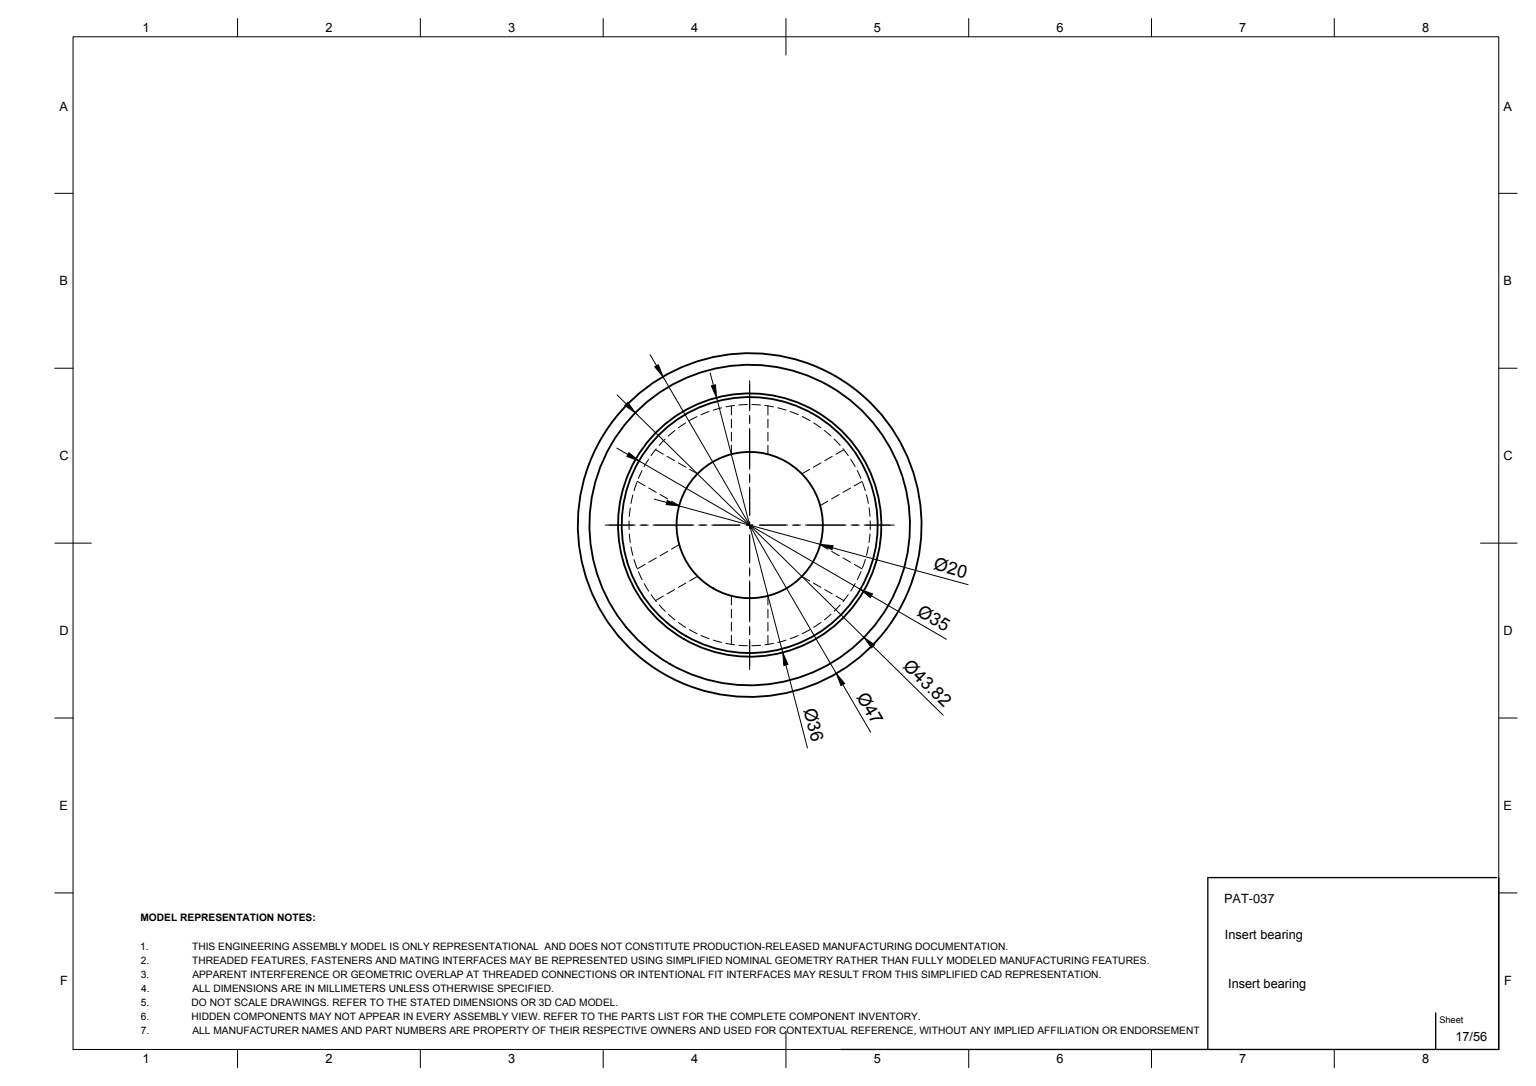
ISO-10303-21;
HEADER;
/* Generated by software containing ST-Developer
 * from STEP Tools, Inc. (www.steptools.com) 
 */

FILE_DESCRIPTION(
/* description */ ('Flywheel Crank-Slider'),
/* implementation_level */ '2;1');

FILE_NAME(
/* name */ 'Insert bearing.step',
/* time_stamp */ '2026-10-28T03:23:13-07:00',
/* author */ (''),
/* organization */ (''),
/* preprocessor_version */ 'ST-DEVELOPER v20.2',
/* originating_system */ 'Autodesk Translation Framework v15.17.0.0',
/* authorisation */ '');

FILE_SCHEMA (('AUTOMOTIVE_DESIGN { 1 0 10303 214 3 1 1 }'));
ENDSEC;

DATA;
#10=MECHANICAL_DESIGN_GEOMETRIC_PRESENTATION_REPRESENTATION('',(#681,#682),#17322);
#457=B_SPLINE_CURVE_WITH_KNOTS('',3,(#14534,#14535,#14536,#14537,#14538,
#14539,#14540,#14541,#14542,#14543),.UNSPECIFIED.,.F.,.F.,(4,2,2,2,4),(1.13193471301885,
1.22626174930539,1.32058878559194,1.41491753480854,1.50924628402513),
 .UNSPECIFIED.);
#458=B_SPLINE_CURVE_WITH_KNOTS('',3,(#14545,#14546,#14547,#14548,#14549,
#14550,#14551,#14552,#14553,#14554,#14555,#14556,#14557,#14558,#14559,#14560,
#14561,#14562),.UNSPECIFIED.,.F.,.F.,(4,2,2,2,2,2,2,2,4),(0.377311571006283,
0.471638607292829,0.565965643579376,0.66029439279597,0.754623142012565,
0.84895189122916,0.943280640445754,1.0376076767323,1.13193471301885),
 .UNSPECIFIED.);
#459=B_SPLINE_CURVE_WITH_KNOTS('',3,(#14563,#14564,#14565,#14566,#14567,
#14568,#14569,#14570,#14571,#14572),.UNSPECIFIED.,.F.,.F.,(4,2,2,2,4),(1.50924628402513,
1.60357503324173,1.69790378245832,1.79223081874487,1.88655785503141),
 .UNSPECIFIED.);
#460=B_SPLINE_CURVE_WITH_KNOTS('',3,(#14575,#14576,#14577,#14578,#14579,
#14580,#14581,#14582,#14583,#14584,#14585,#14586,#14587,#14588,#14589,#14590,
#14591,#14592,#14593,#14594,#14595,#14596,#14597,#14598,#14599,#14600,#14601,
#14602,#14603,#14604,#14605,#14606,#14607,#14608),.UNSPECIFIED.,.T.,.F.,
(4,2,2,2,2,2,2,2,2,2,2,2,2,2,2,2,4),(0.,0.0946120580087934,0.189224116017587,
0.283822945575014,0.378421775132442,0.47302060468987,0.567619434247297,
0.662231492256091,0.756843550264884,0.851455608273677,0.94606766628247,
1.0406664958399,1.13526532539733,1.22986415495475,1.32446298451218,1.41907504252097,
1.51368710052977),.UNSPECIFIED.);
#461=B_SPLINE_CURVE_WITH_KNOTS('',3,(#14611,#14612,#14613,#14614,#14615,
#14616,#14617,#14618,#14619,#14620,#14621,#14622,#14623,#14624,#14625,#14626,
#14627,#14628,#14629,#14630,#14631,#14632,#14633,#14634,#14635,#14636,#14637,
#14638,#14639,#14640,#14641,#14642,#14643,#14644),.UNSPECIFIED.,.T.,.F.,
(4,2,2,2,2,2,2,2,2,2,2,2,2,2,2,2,4),(0.,0.0946120580087934,0.189224116017587,
0.283822945575014,0.378421775132442,0.47302060468987,0.567619434247297,
0.66223149225609,0.756843550264884,0.851455608273677,0.94606766628247,1.0406664958399,
1.13526532539733,1.22986415495475,1.32446298451218,1.41907504252097,1.51368710052977),
 .UNSPECIFIED.);
#462=B_SPLINE_CURVE_WITH_KNOTS('',3,(#14648,#14649,#14650,#14651,#14652,
#14653,#14654,#14655,#14656,#14657),.UNSPECIFIED.,.F.,.F.,(4,2,2,2,4),(1.13193471301885,
1.22626174930539,1.32058878559194,1.41491753480854,1.50924628402513),
 .UNSPECIFIED.);
#463=B_SPLINE_CURVE_WITH_KNOTS('',3,(#14659,#14660,#14661,#14662,#14663,
#14664,#14665,#14666,#14667,#14668,#14669,#14670,#14671,#14672,#14673,#14674,
#14675,#14676),.UNSPECIFIED.,.F.,.F.,(4,2,2,2,2,2,2,2,4),(0.377311571006283,
0.47163860729283,0.565965643579376,0.660294392795971,0.754623142012565,
0.84895189122916,0.943280640445755,1.0376076767323,1.13193471301885),
 .UNSPECIFIED.);
#464=B_SPLINE_CURVE_WITH_KNOTS('',3,(#14677,#14678,#14679,#14680,#14681,
#14682,#14683,#14684,#14685,#14686),.UNSPECIFIED.,.F.,.F.,(4,2,2,2,4),(1.50924628402513,
1.60357503324173,1.69790378245832,1.79223081874487,1.88655785503141),
 .UNSPECIFIED.);
#465=B_SPLINE_CURVE_WITH_KNOTS('',3,(#14695,#14696,#14697,#14698,#14699,
#14700,#14701,#14702,#14703,#14704,#14705,#14706,#14707,#14708,#14709,#14710,
#14711,#14712),.UNSPECIFIED.,.F.,.F.,(4,2,2,2,2,2,2,2,4),(0.377311571006282,
0.471638607292829,0.565965643579376,0.660294392795971,0.754623142012565,
0.84895189122916,0.943280640445754,1.0376076767323,1.13193471301885),
 .UNSPECIFIED.);
#466=B_SPLINE_CURVE_WITH_KNOTS('',3,(#14714,#14715,#14716,#14717,#14718,
#14719,#14720,#14721,#14722,#14723),.UNSPECIFIED.,.F.,.F.,(4,2,2,2,4),(1.13193471301885,
1.22626174930539,1.32058878559194,1.41491753480854,1.50924628402513),
 .UNSPECIFIED.);
#467=B_SPLINE_CURVE_WITH_KNOTS('',3,(#14724,#14725,#14726,#14727,#14728,
#14729,#14730,#14731,#14732,#14733),.UNSPECIFIED.,.F.,.F.,(4,2,2,2,4),(1.50924628402513,
1.60357503324172,1.69790378245832,1.79223081874487,1.88655785503141),
 .UNSPECIFIED.);
#468=B_SPLINE_CURVE_WITH_KNOTS('',3,(#14736,#14737,#14738,#14739,#14740,
#14741,#14742,#14743,#14744,#14745,#14746,#14747,#14748,#14749,#14750,#14751,
#14752,#14753),.UNSPECIFIED.,.F.,.F.,(4,2,2,2,2,2,2,2,4),(0.377311571006283,
0.47163860729283,0.565965643579376,0.660294392795971,0.754623142012565,
0.84895189122916,0.943280640445754,1.0376076767323,1.13193471301885),
 .UNSPECIFIED.);
#469=B_SPLINE_CURVE_WITH_KNOTS('',3,(#14755,#14756,#14757,#14758,#14759,
#14760,#14761,#14762,#14763,#14764),.UNSPECIFIED.,.F.,.F.,(4,2,2,2,4),(1.13193471301885,
1.22626174930539,1.32058878559194,1.41491753480854,1.50924628402513),
 .UNSPECIFIED.);
#470=B_SPLINE_CURVE_WITH_KNOTS('',3,(#14765,#14766,#14767,#14768,#14769,
#14770,#14771,#14772,#14773,#14774),.UNSPECIFIED.,.F.,.F.,(4,2,2,2,4),(1.50924628402513,
1.60357503324173,1.69790378245832,1.79223081874487,1.88655785503141),
 .UNSPECIFIED.);
#471=B_SPLINE_CURVE_WITH_KNOTS('',3,(#14777,#14778,#14779,#14780,#14781,
#14782,#14783,#14784,#14785,#14786,#14787,#14788,#14789,#14790,#14791,#14792,
#14793,#14794),.UNSPECIFIED.,.F.,.F.,(4,2,2,2,2,2,2,2,4),(0.377311571006282,
0.471638607292829,0.565965643579376,0.66029439279597,0.754623142012565,
0.84895189122916,0.943280640445754,1.0376076767323,1.13193471301885),
 .UNSPECIFIED.);
#472=B_SPLINE_CURVE_WITH_KNOTS('',3,(#14796,#14797,#14798,#14799,#14800,
#14801,#14802,#14803,#14804,#14805),.UNSPECIFIED.,.F.,.F.,(4,2,2,2,4),(1.13193471301885,
1.22626174930539,1.32058878559194,1.41491753480854,1.50924628402513),
 .UNSPECIFIED.);
#473=B_SPLINE_CURVE_WITH_KNOTS('',3,(#14806,#14807,#14808,#14809,#14810,
#14811,#14812,#14813,#14814,#14815),.UNSPECIFIED.,.F.,.F.,(4,2,2,2,4),(1.50924628402513,
1.60357503324172,1.69790378245832,1.79223081874487,1.88655785503141),
 .UNSPECIFIED.);
#474=B_SPLINE_CURVE_WITH_KNOTS('',3,(#14818,#14819,#14820,#14821,#14822,
#14823,#14824,#14825,#14826,#14827,#14828,#14829,#14830,#14831,#14832,#14833,
#14834,#14835),.UNSPECIFIED.,.F.,.F.,(4,2,2,2,2,2,2,2,4),(0.377311571006283,
0.471638607292829,0.565965643579376,0.660294392795971,0.754623142012565,
0.84895189122916,0.943280640445755,1.0376076767323,1.13193471301885),
 .UNSPECIFIED.);
#475=B_SPLINE_CURVE_WITH_KNOTS('',3,(#14837,#14838,#14839,#14840,#14841,
#14842,#14843,#14844,#14845,#14846),.UNSPECIFIED.,.F.,.F.,(4,2,2,2,4),(1.13193471301885,
1.22626174930539,1.32058878559194,1.41491753480854,1.50924628402513),
 .UNSPECIFIED.);
#476=B_SPLINE_CURVE_WITH_KNOTS('',3,(#14847,#14848,#14849,#14850,#14851,
#14852,#14853,#14854,#14855,#14856),.UNSPECIFIED.,.F.,.F.,(4,2,2,2,4),(1.50924628402513,
1.60357503324172,1.69790378245832,1.79223081874487,1.88655785503141),
 .UNSPECIFIED.);
#477=B_SPLINE_CURVE_WITH_KNOTS('',3,(#14860,#14861,#14862,#14863,#14864,
#14865,#14866,#14867,#14868,#14869,#14870,#14871,#14872,#14873,#14874,#14875,
#14876,#14877,#14878,#14879,#14880,#14881,#14882,#14883,#14884,#14885,#14886,
#14887,#14888,#14889,#14890,#14891,#14892,#14893),.UNSPECIFIED.,.T.,.F.,
(4,2,2,2,2,2,2,2,2,2,2,2,2,2,2,2,4),(0.,0.0946120580087934,0.189224116017587,
0.283822945575014,0.378421775132442,0.47302060468987,0.567619434247297,
0.66223149225609,0.756843550264884,0.851455608273677,0.94606766628247,1.0406664958399,
1.13526532539733,1.22986415495475,1.32446298451218,1.41907504252097,1.51368710052977),
 .UNSPECIFIED.);
#478=B_SPLINE_CURVE_WITH_KNOTS('',3,(#14896,#14897,#14898,#14899,#14900,
#14901,#14902,#14903,#14904,#14905,#14906,#14907,#14908,#14909,#14910,#14911,
#14912,#14913,#14914,#14915,#14916,#14917,#14918,#14919,#14920,#14921,#14922,
#14923,#14924,#14925,#14926,#14927,#14928,#14929),.UNSPECIFIED.,.T.,.F.,
(4,2,2,2,2,2,2,2,2,2,2,2,2,2,2,2,4),(0.,0.0946120580087934,0.189224116017587,
0.283822945575014,0.378421775132442,0.47302060468987,0.567619434247297,
0.66223149225609,0.756843550264884,0.851455608273677,0.94606766628247,1.0406664958399,
1.13526532539733,1.22986415495475,1.32446298451218,1.41907504252097,1.51368710052977),
 .UNSPECIFIED.);
#479=B_SPLINE_CURVE_WITH_KNOTS('',3,(#14934,#14935,#14936,#14937,#14938,
#14939,#14940,#14941,#14942,#14943,#14944,#14945,#14946,#14947,#14948,#14949,
#14950,#14951,#14952,#14953,#14954,#14955,#14956,#14957,#14958,#14959,#14960,
#14961,#14962,#14963,#14964,#14965,#14966,#14967),.UNSPECIFIED.,.T.,.F.,
(4,2,2,2,2,2,2,2,2,2,2,2,2,2,2,2,4),(0.,0.0946120580087934,0.189224116017587,
0.283822945575014,0.378421775132442,0.47302060468987,0.567619434247297,
0.66223149225609,0.756843550264884,0.851455608273677,0.94606766628247,1.0406664958399,
1.13526532539733,1.22986415495475,1.32446298451218,1.41907504252097,1.51368710052977),
 .UNSPECIFIED.);
#480=B_SPLINE_CURVE_WITH_KNOTS('',3,(#14970,#14971,#14972,#14973,#14974,
#14975,#14976,#14977,#14978,#14979,#14980,#14981,#14982,#14983,#14984,#14985,
#14986,#14987,#14988,#14989,#14990,#14991,#14992,#14993,#14994,#14995,#14996,
#14997,#14998,#14999,#15000,#15001,#15002,#15003),.UNSPECIFIED.,.T.,.F.,
(4,2,2,2,2,2,2,2,2,2,2,2,2,2,2,2,4),(0.,0.0946120580087934,0.189224116017587,
0.283822945575014,0.378421775132442,0.47302060468987,0.567619434247297,
0.66223149225609,0.756843550264884,0.851455608273677,0.94606766628247,1.0406664958399,
1.13526532539733,1.22986415495475,1.32446298451218,1.41907504252097,1.51368710052977),
 .UNSPECIFIED.);
#512=SPHERICAL_SURFACE('',#10020,2.35);
#577=SHAPE_REPRESENTATION_RELATIONSHIP('SRR','None',#17574,#629);
#629=ADVANCED_BREP_SHAPE_REPRESENTATION('',(#741,#742),#17278);
#681=STYLED_ITEM('',(#17931),#741);
#682=STYLED_ITEM('',(#17931),#742);
#741=MANIFOLD_SOLID_BREP('Body1',#9060);
#742=MANIFOLD_SOLID_BREP('Body2',#9061);
#872=FACE_BOUND('',#2118,.T.);
#873=FACE_BOUND('',#2120,.T.);
#874=FACE_BOUND('',#2121,.T.);
#875=FACE_BOUND('',#2123,.T.);
#876=FACE_BOUND('',#2127,.T.);
#877=FACE_BOUND('',#2128,.T.);
#878=FACE_BOUND('',#2129,.T.);
#879=FACE_BOUND('',#2130,.T.);
#880=FACE_BOUND('',#2131,.T.);
#881=FACE_BOUND('',#2132,.T.);
#882=FACE_BOUND('',#2138,.T.);
#883=FACE_BOUND('',#2140,.T.);
#884=FACE_BOUND('',#2143,.T.);
#885=FACE_BOUND('',#2145,.T.);
#886=FACE_BOUND('',#2146,.T.);
#887=FACE_BOUND('',#2147,.T.);
#888=FACE_BOUND('',#2148,.T.);
#889=FACE_BOUND('',#2149,.T.);
#890=FACE_BOUND('',#2150,.T.);
#1115=PLANE('',#10018);
#1116=PLANE('',#10023);
#1117=PLANE('',#10033);
#1118=PLANE('',#10035);
#1119=PLANE('',#10039);
#1494=FACE_OUTER_BOUND('',#2116,.T.);
#1495=FACE_OUTER_BOUND('',#2117,.T.);
#1496=FACE_OUTER_BOUND('',#2119,.T.);
#1497=FACE_OUTER_BOUND('',#2122,.T.);
#1498=FACE_OUTER_BOUND('',#2124,.T.);
#1499=FACE_OUTER_BOUND('',#2125,.T.);
#1500=FACE_OUTER_BOUND('',#2126,.T.);
#1501=FACE_OUTER_BOUND('',#2133,.T.);
#1502=FACE_OUTER_BOUND('',#2134,.T.);
#1503=FACE_OUTER_BOUND('',#2135,.T.);
#1504=FACE_OUTER_BOUND('',#2136,.T.);
#1505=FACE_OUTER_BOUND('',#2137,.T.);
#1506=FACE_OUTER_BOUND('',#2139,.T.);
#1507=FACE_OUTER_BOUND('',#2141,.T.);
#1508=FACE_OUTER_BOUND('',#2142,.T.);
#1509=FACE_OUTER_BOUND('',#2144,.T.);
#2116=EDGE_LOOP('',(#6840,#6841,#6842,#6843));
#2117=EDGE_LOOP('',(#6844));
#2118=EDGE_LOOP('',(#6845));
#2119=EDGE_LOOP('',(#6846,#6847));
#2120=EDGE_LOOP('',(#6848));
#2121=EDGE_LOOP('',(#6849));
#2122=EDGE_LOOP('',(#6850));
#2123=EDGE_LOOP('',(#6851));
#2124=EDGE_LOOP('',(#6852,#6853,#6854,#6855,#6856,#6857));
#2125=EDGE_LOOP('',(#6858,#6859,#6860,#6861,#6862,#6863));
#2126=EDGE_LOOP('',(#6864,#6865,#6866,#6867));
#2127=EDGE_LOOP('',(#6868,#6869,#6870));
#2128=EDGE_LOOP('',(#6871,#6872,#6873));
#2129=EDGE_LOOP('',(#6874,#6875,#6876));
#2130=EDGE_LOOP('',(#6877,#6878,#6879));
#2131=EDGE_LOOP('',(#6880,#6881,#6882));
#2132=EDGE_LOOP('',(#6883,#6884,#6885));
#2133=EDGE_LOOP('',(#6886,#6887,#6888,#6889,#6890,#6891));
#2134=EDGE_LOOP('',(#6892,#6893,#6894,#6895,#6896,#6897));
#2135=EDGE_LOOP('',(#6898,#6899,#6900,#6901,#6902,#6903));
#2136=EDGE_LOOP('',(#6904,#6905,#6906,#6907,#6908,#6909));
#2137=EDGE_LOOP('',(#6910));
#2138=EDGE_LOOP('',(#6911));
#2139=EDGE_LOOP('',(#6912));
#2140=EDGE_LOOP('',(#6913));
#2141=EDGE_LOOP('',(#6914,#6915,#6916,#6917));
#2142=EDGE_LOOP('',(#6918));
#2143=EDGE_LOOP('',(#6919));
#2144=EDGE_LOOP('',(#6920,#6921,#6922,#6923));
#2145=EDGE_LOOP('',(#6924));
#2146=EDGE_LOOP('',(#6925));
#2147=EDGE_LOOP('',(#6926));
#2148=EDGE_LOOP('',(#6927));
#2149=EDGE_LOOP('',(#6928));
#2150=EDGE_LOOP('',(#6929));
#2836=LINE('',#14519,#3447);
#2837=LINE('',#14574,#3448);
#2838=LINE('',#14646,#3449);
#2839=LINE('',#14691,#3450);
#2840=LINE('',#14859,#3451);
#2841=LINE('',#14930,#3452);
#2842=LINE('',#14933,#3453);
#2843=LINE('',#15004,#3454);
#2844=LINE('',#15014,#3455);
#2845=LINE('',#15019,#3456);
#3447=VECTOR('',#11714,1.8);
#3448=VECTOR('',#11731,0.25);
#3449=VECTOR('',#11734,0.25);
#3450=VECTOR('',#11739,1.65);
#3451=VECTOR('',#11744,0.25);
#3452=VECTOR('',#11747,0.25);
#3453=VECTOR('',#11750,0.25);
#3454=VECTOR('',#11753,0.25);
#3455=VECTOR('',#11766,1.75);
#3456=VECTOR('',#11773,1.);
#3977=CIRCLE('',#10016,1.8);
#3978=CIRCLE('',#10017,1.8);
#3979=CIRCLE('',#10019,2.19089023002066);
#3980=CIRCLE('',#10021,2.35);
#3981=CIRCLE('',#10022,2.19089023002066);
#3982=CIRCLE('',#10027,1.65);
#3983=CIRCLE('',#10028,1.65);
#3984=CIRCLE('',#10034,1.);
#3985=CIRCLE('',#10036,1.75);
#3986=CIRCLE('',#10038,1.75);
#3987=CIRCLE('',#10040,1.);
#4511=VERTEX_POINT('',#14516);
#4512=VERTEX_POINT('',#14518);
#4513=VERTEX_POINT('',#14522);
#4514=VERTEX_POINT('',#14525);
#4515=VERTEX_POINT('',#14526);
#4516=VERTEX_POINT('',#14528);
#4517=VERTEX_POINT('',#14532);
#4518=VERTEX_POINT('',#14533);
#4519=VERTEX_POINT('',#14544);
#4520=VERTEX_POINT('',#14573);
#4521=VERTEX_POINT('',#14610);
#4522=VERTEX_POINT('',#14645);
#4523=VERTEX_POINT('',#14647);
#4524=VERTEX_POINT('',#14658);
#4525=VERTEX_POINT('',#14688);
#4526=VERTEX_POINT('',#14690);
#4527=VERTEX_POINT('',#14693);
#4528=VERTEX_POINT('',#14694);
#4529=VERTEX_POINT('',#14713);
#4530=VERTEX_POINT('',#14734);
#4531=VERTEX_POINT('',#14735);
#4532=VERTEX_POINT('',#14754);
#4533=VERTEX_POINT('',#14775);
#4534=VERTEX_POINT('',#14776);
#4535=VERTEX_POINT('',#14795);
#4536=VERTEX_POINT('',#14816);
#4537=VERTEX_POINT('',#14817);
#4538=VERTEX_POINT('',#14836);
#4539=VERTEX_POINT('',#14858);
#4540=VERTEX_POINT('',#14895);
#4541=VERTEX_POINT('',#14932);
#4542=VERTEX_POINT('',#14969);
#4543=VERTEX_POINT('',#15006);
#4544=VERTEX_POINT('',#15009);
#4545=VERTEX_POINT('',#15012);
#4546=VERTEX_POINT('',#15016);
#5377=EDGE_CURVE('',#4511,#4511,#3977,.T.);
#5378=EDGE_CURVE('',#4511,#4512,#2836,.T.);
#5379=EDGE_CURVE('',#4512,#4512,#3978,.T.);
#5380=EDGE_CURVE('',#4513,#4513,#3979,.T.);
#5381=EDGE_CURVE('',#4514,#4515,#3980,.T.);
#5382=EDGE_CURVE('',#4516,#4516,#3981,.T.);
#5383=EDGE_CURVE('',#4517,#4518,#457,.T.);
#5384=EDGE_CURVE('',#4519,#4517,#458,.T.);
#5385=EDGE_CURVE('',#4518,#4519,#459,.T.);
#5386=EDGE_CURVE('',#4518,#4520,#2837,.T.);
#5387=EDGE_CURVE('',#4520,#4520,#460,.T.);
#5388=EDGE_CURVE('',#4521,#4521,#461,.T.);
#5389=EDGE_CURVE('',#4521,#4522,#2838,.T.);
#5390=EDGE_CURVE('',#4523,#4522,#462,.T.);
#5391=EDGE_CURVE('',#4524,#4523,#463,.T.);
#5392=EDGE_CURVE('',#4522,#4524,#464,.T.);
#5393=EDGE_CURVE('',#4525,#4525,#3982,.T.);
#5394=EDGE_CURVE('',#4525,#4526,#2839,.T.);
#5395=EDGE_CURVE('',#4526,#4526,#3983,.T.);
#5396=EDGE_CURVE('',#4527,#4528,#465,.T.);
#5397=EDGE_CURVE('',#4528,#4529,#466,.T.);
#5398=EDGE_CURVE('',#4529,#4527,#467,.T.);
#5399=EDGE_CURVE('',#4530,#4531,#468,.T.);
#5400=EDGE_CURVE('',#4531,#4532,#469,.T.);
#5401=EDGE_CURVE('',#4532,#4530,#470,.T.);
#5402=EDGE_CURVE('',#4533,#4534,#471,.T.);
#5403=EDGE_CURVE('',#4534,#4535,#472,.T.);
#5404=EDGE_CURVE('',#4535,#4533,#473,.T.);
#5405=EDGE_CURVE('',#4536,#4537,#474,.T.);
#5406=EDGE_CURVE('',#4537,#4538,#475,.T.);
#5407=EDGE_CURVE('',#4538,#4536,#476,.T.);
#5408=EDGE_CURVE('',#4529,#4539,#2840,.T.);
#5409=EDGE_CURVE('',#4539,#4539,#477,.T.);
#5410=EDGE_CURVE('',#4540,#4540,#478,.T.);
#5411=EDGE_CURVE('',#4540,#4532,#2841,.T.);
#5412=EDGE_CURVE('',#4535,#4541,#2842,.T.);
#5413=EDGE_CURVE('',#4541,#4541,#479,.T.);
#5414=EDGE_CURVE('',#4542,#4542,#480,.T.);
#5415=EDGE_CURVE('',#4542,#4538,#2843,.T.);
#5416=EDGE_CURVE('',#4543,#4543,#3984,.T.);
#5417=EDGE_CURVE('',#4544,#4544,#3985,.T.);
#5418=EDGE_CURVE('',#4545,#4545,#3986,.T.);
#5419=EDGE_CURVE('',#4545,#4544,#2844,.T.);
#5420=EDGE_CURVE('',#4546,#4546,#3987,.T.);
#5421=EDGE_CURVE('',#4546,#4543,#2845,.T.);
#6840=ORIENTED_EDGE('',*,*,#5377,.T.);
#6841=ORIENTED_EDGE('',*,*,#5378,.T.);
#6842=ORIENTED_EDGE('',*,*,#5379,.F.);
#6843=ORIENTED_EDGE('',*,*,#5378,.F.);
#6844=ORIENTED_EDGE('',*,*,#5380,.F.);
#6845=ORIENTED_EDGE('',*,*,#5379,.T.);
#6846=ORIENTED_EDGE('',*,*,#5381,.T.);
#6847=ORIENTED_EDGE('',*,*,#5381,.F.);
#6848=ORIENTED_EDGE('',*,*,#5380,.T.);
#6849=ORIENTED_EDGE('',*,*,#5382,.F.);
#6850=ORIENTED_EDGE('',*,*,#5382,.T.);
#6851=ORIENTED_EDGE('',*,*,#5377,.F.);
#6852=ORIENTED_EDGE('',*,*,#5383,.F.);
#6853=ORIENTED_EDGE('',*,*,#5384,.F.);
#6854=ORIENTED_EDGE('',*,*,#5385,.F.);
#6855=ORIENTED_EDGE('',*,*,#5386,.T.);
#6856=ORIENTED_EDGE('',*,*,#5387,.F.);
#6857=ORIENTED_EDGE('',*,*,#5386,.F.);
#6858=ORIENTED_EDGE('',*,*,#5388,.F.);
#6859=ORIENTED_EDGE('',*,*,#5389,.T.);
#6860=ORIENTED_EDGE('',*,*,#5390,.F.);
#6861=ORIENTED_EDGE('',*,*,#5391,.F.);
#6862=ORIENTED_EDGE('',*,*,#5392,.F.);
#6863=ORIENTED_EDGE('',*,*,#5389,.F.);
#6864=ORIENTED_EDGE('',*,*,#5393,.F.);
#6865=ORIENTED_EDGE('',*,*,#5394,.T.);
#6866=ORIENTED_EDGE('',*,*,#5395,.T.);
#6867=ORIENTED_EDGE('',*,*,#5394,.F.);
#6868=ORIENTED_EDGE('',*,*,#5384,.T.);
#6869=ORIENTED_EDGE('',*,*,#5383,.T.);
#6870=ORIENTED_EDGE('',*,*,#5385,.T.);
#6871=ORIENTED_EDGE('',*,*,#5391,.T.);
#6872=ORIENTED_EDGE('',*,*,#5390,.T.);
#6873=ORIENTED_EDGE('',*,*,#5392,.T.);
#6874=ORIENTED_EDGE('',*,*,#5396,.T.);
#6875=ORIENTED_EDGE('',*,*,#5397,.T.);
#6876=ORIENTED_EDGE('',*,*,#5398,.T.);
#6877=ORIENTED_EDGE('',*,*,#5399,.T.);
#6878=ORIENTED_EDGE('',*,*,#5400,.T.);
#6879=ORIENTED_EDGE('',*,*,#5401,.T.);
#6880=ORIENTED_EDGE('',*,*,#5402,.T.);
#6881=ORIENTED_EDGE('',*,*,#5403,.T.);
#6882=ORIENTED_EDGE('',*,*,#5404,.T.);
#6883=ORIENTED_EDGE('',*,*,#5405,.T.);
#6884=ORIENTED_EDGE('',*,*,#5406,.T.);
#6885=ORIENTED_EDGE('',*,*,#5407,.T.);
#6886=ORIENTED_EDGE('',*,*,#5397,.F.);
#6887=ORIENTED_EDGE('',*,*,#5396,.F.);
#6888=ORIENTED_EDGE('',*,*,#5398,.F.);
#6889=ORIENTED_EDGE('',*,*,#5408,.T.);
#6890=ORIENTED_EDGE('',*,*,#5409,.F.);
#6891=ORIENTED_EDGE('',*,*,#5408,.F.);
#6892=ORIENTED_EDGE('',*,*,#5410,.F.);
#6893=ORIENTED_EDGE('',*,*,#5411,.T.);
#6894=ORIENTED_EDGE('',*,*,#5400,.F.);
#6895=ORIENTED_EDGE('',*,*,#5399,.F.);
#6896=ORIENTED_EDGE('',*,*,#5401,.F.);
#6897=ORIENTED_EDGE('',*,*,#5411,.F.);
#6898=ORIENTED_EDGE('',*,*,#5403,.F.);
#6899=ORIENTED_EDGE('',*,*,#5402,.F.);
#6900=ORIENTED_EDGE('',*,*,#5404,.F.);
#6901=ORIENTED_EDGE('',*,*,#5412,.T.);
#6902=ORIENTED_EDGE('',*,*,#5413,.F.);
#6903=ORIENTED_EDGE('',*,*,#5412,.F.);
#6904=ORIENTED_EDGE('',*,*,#5414,.F.);
#6905=ORIENTED_EDGE('',*,*,#5415,.T.);
#6906=ORIENTED_EDGE('',*,*,#5406,.F.);
#6907=ORIENTED_EDGE('',*,*,#5405,.F.);
#6908=ORIENTED_EDGE('',*,*,#5407,.F.);
#6909=ORIENTED_EDGE('',*,*,#5415,.F.);
#6910=ORIENTED_EDGE('',*,*,#5395,.F.);
#6911=ORIENTED_EDGE('',*,*,#5416,.T.);
#6912=ORIENTED_EDGE('',*,*,#5417,.F.);
#6913=ORIENTED_EDGE('',*,*,#5393,.T.);
#6914=ORIENTED_EDGE('',*,*,#5418,.F.);
#6915=ORIENTED_EDGE('',*,*,#5419,.T.);
#6916=ORIENTED_EDGE('',*,*,#5417,.T.);
#6917=ORIENTED_EDGE('',*,*,#5419,.F.);
#6918=ORIENTED_EDGE('',*,*,#5418,.T.);
#6919=ORIENTED_EDGE('',*,*,#5420,.F.);
#6920=ORIENTED_EDGE('',*,*,#5420,.T.);
#6921=ORIENTED_EDGE('',*,*,#5421,.T.);
#6922=ORIENTED_EDGE('',*,*,#5416,.F.);
#6923=ORIENTED_EDGE('',*,*,#5421,.F.);
#6924=ORIENTED_EDGE('',*,*,#5388,.T.);
#6925=ORIENTED_EDGE('',*,*,#5387,.T.);
#6926=ORIENTED_EDGE('',*,*,#5410,.T.);
#6927=ORIENTED_EDGE('',*,*,#5409,.T.);
#6928=ORIENTED_EDGE('',*,*,#5414,.T.);
#6929=ORIENTED_EDGE('',*,*,#5413,.T.);
#8395=CYLINDRICAL_SURFACE('',#10015,1.8);
#8396=CYLINDRICAL_SURFACE('',#10024,0.25);
#8397=CYLINDRICAL_SURFACE('',#10025,0.25);
#8398=CYLINDRICAL_SURFACE('',#10026,1.65);
#8399=CYLINDRICAL_SURFACE('',#10029,0.25);
#8400=CYLINDRICAL_SURFACE('',#10030,0.25);
#8401=CYLINDRICAL_SURFACE('',#10031,0.25);
#8402=CYLINDRICAL_SURFACE('',#10032,0.25);
#8403=CYLINDRICAL_SURFACE('',#10037,1.75);
#8404=CYLINDRICAL_SURFACE('',#10041,1.);
#8685=ADVANCED_FACE('',(#1494),#8395,.F.);
#8686=ADVANCED_FACE('',(#1495,#872),#1115,.T.);
#8687=ADVANCED_FACE('',(#1496,#873,#874),#512,.T.);
#8688=ADVANCED_FACE('',(#1497,#875),#1116,.T.);
#8689=ADVANCED_FACE('',(#1498),#8396,.F.);
#8690=ADVANCED_FACE('',(#1499),#8397,.F.);
#8691=ADVANCED_FACE('',(#1500,#876,#877,#878,#879,#880,#881),#8398,.T.);
#8692=ADVANCED_FACE('',(#1501),#8399,.F.);
#8693=ADVANCED_FACE('',(#1502),#8400,.F.);
#8694=ADVANCED_FACE('',(#1503),#8401,.F.);
#8695=ADVANCED_FACE('',(#1504),#8402,.F.);
#8696=ADVANCED_FACE('',(#1505,#882),#1117,.T.);
#8697=ADVANCED_FACE('',(#1506,#883),#1118,.T.);
#8698=ADVANCED_FACE('',(#1507),#8403,.T.);
#8699=ADVANCED_FACE('',(#1508,#884),#1119,.T.);
#8700=ADVANCED_FACE('',(#1509,#885,#886,#887,#888,#889,#890),#8404,.F.);
#9060=CLOSED_SHELL('',(#8685,#8686,#8687,#8688));
#9061=CLOSED_SHELL('',(#8689,#8690,#8691,#8692,#8693,#8694,#8695,#8696,
#8697,#8698,#8699,#8700));
#10014=AXIS2_PLACEMENT_3D('',#14514,#11708,#11709);
#10015=AXIS2_PLACEMENT_3D('',#14515,#11710,#11711);
#10016=AXIS2_PLACEMENT_3D('',#14517,#11712,#11713);
#10017=AXIS2_PLACEMENT_3D('',#14520,#11715,#11716);
#10018=AXIS2_PLACEMENT_3D('',#14521,#11717,#11718);
#10019=AXIS2_PLACEMENT_3D('',#14523,#11719,#11720);
#10020=AXIS2_PLACEMENT_3D('',#14524,#11721,#11722);
#10021=AXIS2_PLACEMENT_3D('',#14527,#11723,#11724);
#10022=AXIS2_PLACEMENT_3D('',#14529,#11725,#11726);
#10023=AXIS2_PLACEMENT_3D('',#14530,#11727,#11728);
#10024=AXIS2_PLACEMENT_3D('',#14531,#11729,#11730);
#10025=AXIS2_PLACEMENT_3D('',#14609,#11732,#11733);
#10026=AXIS2_PLACEMENT_3D('',#14687,#11735,#11736);
#10027=AXIS2_PLACEMENT_3D('',#14689,#11737,#11738);
#10028=AXIS2_PLACEMENT_3D('',#14692,#11740,#11741);
#10029=AXIS2_PLACEMENT_3D('',#14857,#11742,#11743);
#10030=AXIS2_PLACEMENT_3D('',#14894,#11745,#11746);
#10031=AXIS2_PLACEMENT_3D('',#14931,#11748,#11749);
#10032=AXIS2_PLACEMENT_3D('',#14968,#11751,#11752);
#10033=AXIS2_PLACEMENT_3D('',#15005,#11754,#11755);
#10034=AXIS2_PLACEMENT_3D('',#15007,#11756,#11757);
#10035=AXIS2_PLACEMENT_3D('',#15008,#11758,#11759);
#10036=AXIS2_PLACEMENT_3D('',#15010,#11760,#11761);
#10037=AXIS2_PLACEMENT_3D('',#15011,#11762,#11763);
#10038=AXIS2_PLACEMENT_3D('',#15013,#11764,#11765);
#10039=AXIS2_PLACEMENT_3D('',#15015,#11767,#11768);
#10040=AXIS2_PLACEMENT_3D('',#15017,#11769,#11770);
#10041=AXIS2_PLACEMENT_3D('',#15018,#11771,#11772);
#11708=DIRECTION('axis',(0.,0.,1.));
#11709=DIRECTION('refdir',(1.,0.,0.));
#11710=DIRECTION('center_axis',(0.,-1.,0.));
#11711=DIRECTION('ref_axis',(1.,0.,0.));
#11712=DIRECTION('center_axis',(0.,-1.,0.));
#11713=DIRECTION('ref_axis',(1.,0.,0.));
#11714=DIRECTION('',(0.,1.,0.));
#11715=DIRECTION('center_axis',(0.,-1.,0.));
#11716=DIRECTION('ref_axis',(1.,0.,0.));
#11717=DIRECTION('center_axis',(0.,1.,0.));
#11718=DIRECTION('ref_axis',(0.,0.,1.));
#11719=DIRECTION('center_axis',(0.,-1.,0.));
#11720=DIRECTION('ref_axis',(1.,0.,0.));
#11721=DIRECTION('center_axis',(6.12323399573677E-17,0.,1.));
#11722=DIRECTION('ref_axis',(1.,0.,0.));
#11723=DIRECTION('center_axis',(1.22464679914735E-16,-1.,0.));
#11724=DIRECTION('ref_axis',(-1.,-1.22464679914735E-16,0.));
#11725=DIRECTION('center_axis',(0.,-1.,0.));
#11726=DIRECTION('ref_axis',(1.,0.,0.));
#11727=DIRECTION('center_axis',(0.,-1.,0.));
#11728=DIRECTION('ref_axis',(0.,0.,-1.));
#11729=DIRECTION('center_axis',(-0.866025403784438,0.,-0.5));
#11730=DIRECTION('ref_axis',(-0.5,0.,0.866025403784438));
#11731=DIRECTION('',(-0.866025403784438,0.,-0.5));
#11732=DIRECTION('center_axis',(-0.866025403784438,0.,-0.5));
#11733=DIRECTION('ref_axis',(-0.5,0.,0.866025403784438));
#11734=DIRECTION('',(-0.866025403784438,0.,-0.5));
#11735=DIRECTION('center_axis',(0.,-1.,0.));
#11736=DIRECTION('ref_axis',(1.,0.,0.));
#11737=DIRECTION('center_axis',(0.,-1.,0.));
#11738=DIRECTION('ref_axis',(1.,0.,0.));
#11739=DIRECTION('',(0.,1.,0.));
#11740=DIRECTION('center_axis',(0.,-1.,0.));
#11741=DIRECTION('ref_axis',(1.,0.,0.));
#11742=DIRECTION('center_axis',(0.866025403784439,0.,-0.5));
#11743=DIRECTION('ref_axis',(-0.5,0.,-0.866025403784439));
#11744=DIRECTION('',(0.866025403784439,0.,-0.5));
#11745=DIRECTION('center_axis',(0.866025403784439,0.,-0.5));
#11746=DIRECTION('ref_axis',(-0.5,0.,-0.866025403784439));
#11747=DIRECTION('',(0.866025403784439,0.,-0.5));
#11748=DIRECTION('center_axis',(0.,0.,1.));
#11749=DIRECTION('ref_axis',(1.,0.,0.));
#11750=DIRECTION('',(0.,0.,1.));
#11751=DIRECTION('center_axis',(0.,0.,1.));
#11752=DIRECTION('ref_axis',(1.,0.,0.));
#11753=DIRECTION('',(0.,0.,1.));
#11754=DIRECTION('center_axis',(0.,1.,0.));
#11755=DIRECTION('ref_axis',(0.,0.,1.));
#11756=DIRECTION('center_axis',(0.,-1.,0.));
#11757=DIRECTION('ref_axis',(1.,0.,0.));
#11758=DIRECTION('center_axis',(0.,1.,0.));
#11759=DIRECTION('ref_axis',(0.,0.,1.));
#11760=DIRECTION('center_axis',(0.,-1.,0.));
#11761=DIRECTION('ref_axis',(1.,0.,0.));
#11762=DIRECTION('center_axis',(0.,-1.,0.));
#11763=DIRECTION('ref_axis',(1.,0.,0.));
#11764=DIRECTION('center_axis',(0.,-1.,0.));
#11765=DIRECTION('ref_axis',(1.,0.,0.));
#11766=DIRECTION('',(0.,1.,0.));
#11767=DIRECTION('center_axis',(0.,-1.,0.));
#11768=DIRECTION('ref_axis',(0.,0.,-1.));
#11769=DIRECTION('center_axis',(0.,-1.,0.));
#11770=DIRECTION('ref_axis',(1.,0.,0.));
#11771=DIRECTION('center_axis',(0.,-1.,0.));
#11772=DIRECTION('ref_axis',(1.,0.,0.));
#11773=DIRECTION('',(0.,1.,0.));
#14514=CARTESIAN_POINT('',(0.,0.,0.));
#14515=CARTESIAN_POINT('Origin',(0.,0.,0.));
#14516=CARTESIAN_POINT('',(-1.8,-0.85,-2.20436423846524E-16));
#14517=CARTESIAN_POINT('Origin',(0.,-0.85,0.));
#14518=CARTESIAN_POINT('',(-1.8,0.85,-2.20436423846524E-16));
#14519=CARTESIAN_POINT('',(-1.8,0.,-2.20436423846524E-16));
#14520=CARTESIAN_POINT('Origin',(0.,0.85,0.));
#14521=CARTESIAN_POINT('Origin',(2.19089023002066,0.85,0.));
#14522=CARTESIAN_POINT('',(2.19089023002066,0.85,0.));
#14523=CARTESIAN_POINT('Origin',(0.,0.85,0.));
#14524=CARTESIAN_POINT('Origin',(3.99680288865056E-15,0.,0.));
#14525=CARTESIAN_POINT('',(3.85290688975075E-15,-1.76221774462768E-32,2.35));
#14526=CARTESIAN_POINT('',(3.85290688975075E-15,-1.76221774462768E-32,-2.35));
#14527=CARTESIAN_POINT('Origin',(3.99680288865056E-15,0.,0.));
#14528=CARTESIAN_POINT('',(2.19089023002066,-0.85,0.));
#14529=CARTESIAN_POINT('Origin',(0.,-0.85,0.));
#14530=CARTESIAN_POINT('Origin',(1.8,-0.85,0.));
#14531=CARTESIAN_POINT('Origin',(0.,1.55,0.));
#14532=CARTESIAN_POINT('',(1.42894191624432,1.8,0.825000000000001));
#14533=CARTESIAN_POINT('',(1.53744468918255,1.55,0.598968970568896));
#14534=CARTESIAN_POINT('Ctrl Pts',(1.42894191624432,1.8,0.825000000000001));
#14535=CARTESIAN_POINT('Ctrl Pts',(1.44466308895875,1.8,0.797770130104052));
#14536=CARTESIAN_POINT('Ctrl Pts',(1.46055812562105,1.79370633789704,0.768258557763732));
#14537=CARTESIAN_POINT('Ctrl Pts',(1.48824888379079,1.76817777258318,0.713138492740816));
#14538=CARTESIAN_POINT('Ctrl Pts',(1.50008999307766,1.74894552961493,0.687551581002689));
#14539=CARTESIAN_POINT('Ctrl Pts',(1.51812136280714,1.70460745840382,0.646764802471699));
#14540=CARTESIAN_POINT('Ctrl Pts',(1.52552758004446,1.67652816181843,0.628833667319578));
#14541=CARTESIAN_POINT('Ctrl Pts',(1.53516661651472,1.61494799959182,0.604921184808251));
#14542=CARTESIAN_POINT('Ctrl Pts',(1.53744468918255,1.58144291640553,0.598968970568896));
#14543=CARTESIAN_POINT('Ctrl Pts',(1.53744468918255,1.55,0.598968970568896));
#14544=CARTESIAN_POINT('',(1.42894191624432,1.3,0.825000000000001));
#14545=CARTESIAN_POINT('Ctrl Pts',(1.42894191624432,1.3,0.825000000000001));
#14546=CARTESIAN_POINT('Ctrl Pts',(1.4132207435299,1.3,0.852229869895949));
#14547=CARTESIAN_POINT('Ctrl Pts',(1.39561049050871,1.30629366210296,0.880751161609749));
#14548=CARTESIAN_POINT('Ctrl Pts',(1.36172049302549,1.33182222741682,0.932292094146256));
#14549=CARTESIAN_POINT('Ctrl Pts',(1.34548213209931,1.35105447038507,0.955340251466734));
#14550=CARTESIAN_POINT('Ctrl Pts',(1.31917543061769,1.39539254159618,0.99134926498299));
#14551=CARTESIAN_POINT('Ctrl Pts',(1.30734972067592,1.42347183818157,1.00672880483252));
#14552=CARTESIAN_POINT('Ctrl Pts',(1.29146042158868,1.48505200040818,1.02703269653942));
#14553=CARTESIAN_POINT('Ctrl Pts',(1.28744468918255,1.51855708359447,1.03198167246111));
#14554=CARTESIAN_POINT('Ctrl Pts',(1.28744468918255,1.58144291640553,1.03198167246111));
#14555=CARTESIAN_POINT('Ctrl Pts',(1.29146042158868,1.61494799959182,1.02703269653942));
#14556=CARTESIAN_POINT('Ctrl Pts',(1.30734972067592,1.67652816181843,1.00672880483252));
#14557=CARTESIAN_POINT('Ctrl Pts',(1.31917543061769,1.70460745840382,0.991349264982991));
#14558=CARTESIAN_POINT('Ctrl Pts',(1.34548213209931,1.74894552961493,0.955340251466735));
#14559=CARTESIAN_POINT('Ctrl Pts',(1.36172049302549,1.76817777258318,0.932292094146256));
#14560=CARTESIAN_POINT('Ctrl Pts',(1.39561049050871,1.79370633789704,0.880751161609749));
#14561=CARTESIAN_POINT('Ctrl Pts',(1.4132207435299,1.8,0.85222986989595));
#14562=CARTESIAN_POINT('Ctrl Pts',(1.42894191624432,1.8,0.825000000000001));
#14563=CARTESIAN_POINT('Ctrl Pts',(1.53744468918255,1.55,0.598968970568896));
#14564=CARTESIAN_POINT('Ctrl Pts',(1.53744468918255,1.51855708359447,0.598968970568896));
#14565=CARTESIAN_POINT('Ctrl Pts',(1.53516661651472,1.48505200040818,0.60492118480825));
#14566=CARTESIAN_POINT('Ctrl Pts',(1.52552758004446,1.42347183818157,0.628833667319578));
#14567=CARTESIAN_POINT('Ctrl Pts',(1.51812136280714,1.39539254159618,0.646764802471699));
#14568=CARTESIAN_POINT('Ctrl Pts',(1.50008999307766,1.35105447038507,0.687551581002689));
#14569=CARTESIAN_POINT('Ctrl Pts',(1.48824888379079,1.33182222741682,0.713138492740816));
#14570=CARTESIAN_POINT('Ctrl Pts',(1.46055812562105,1.30629366210296,0.768258557763732));
#14571=CARTESIAN_POINT('Ctrl Pts',(1.44466308895875,1.3,0.797770130104052));
#14572=CARTESIAN_POINT('Ctrl Pts',(1.42894191624432,1.3,0.825000000000001));
#14573=CARTESIAN_POINT('',(0.963525491562421,1.55,0.267616567329818));
#14574=CARTESIAN_POINT('',(0.125,1.55,-0.21650635094611));
#14575=CARTESIAN_POINT('Ctrl Pts',(0.963525491562421,1.55,0.267616567329818));
#14576=CARTESIAN_POINT('Ctrl Pts',(0.963525491562421,1.5815373526696,0.267616567329818));
#14577=CARTESIAN_POINT('Ctrl Pts',(0.961833761492987,1.61508042700263,0.273949373987484));
#14578=CARTESIAN_POINT('Ctrl Pts',(0.954308486908894,1.67663267125761,0.299111603474268));
#14579=CARTESIAN_POINT('Ctrl Pts',(0.948394987258249,1.70465411363682,0.31788699900678));
#14580=CARTESIAN_POINT('Ctrl Pts',(0.933155485613026,1.74889618382539,0.360174810895352));
#14581=CARTESIAN_POINT('Ctrl Pts',(0.92278792026947,1.76811531482682,0.386546956384144));
#14582=CARTESIAN_POINT('Ctrl Pts',(0.897143218189782,1.79367084275751,0.442820664919227));
#14583=CARTESIAN_POINT('Ctrl Pts',(0.881791875377343,1.8,0.472691670144998));
#14584=CARTESIAN_POINT('Ctrl Pts',(0.850258932191534,1.8,0.527308329855003));
#14585=CARTESIAN_POINT('Ctrl Pts',(0.832065554235658,1.79367084275751,0.555538485325664));
#14586=CARTESIAN_POINT('Ctrl Pts',(0.796153444118959,1.76811531482682,0.605884303066698));
#14587=CARTESIAN_POINT('Ctrl Pts',(0.778498278845144,1.74889618382539,0.62804895077401));
#14588=CARTESIAN_POINT('Ctrl Pts',(0.749495710301794,1.70465411363682,0.662390652284073));
#14589=CARTESIAN_POINT('Ctrl Pts',(0.73619249062986,1.67663267125761,0.676899590973058));
#14590=CARTESIAN_POINT('Ctrl Pts',(0.718163997970498,1.61508042700263,0.695997784676728));
#14591=CARTESIAN_POINT('Ctrl Pts',(0.713525491562421,1.5815373526696,0.700629269222037));
#14592=CARTESIAN_POINT('Ctrl Pts',(0.713525491562421,1.5184626473304,0.700629269222037));
#14593=CARTESIAN_POINT('Ctrl Pts',(0.718163997970498,1.48491957299737,0.695997784676728));
#14594=CARTESIAN_POINT('Ctrl Pts',(0.73619249062986,1.42336732874239,0.676899590973058));
#14595=CARTESIAN_POINT('Ctrl Pts',(0.749495710301794,1.39534588636318,0.662390652284073));
#14596=CARTESIAN_POINT('Ctrl Pts',(0.778498278845144,1.35110381617461,0.62804895077401));
#14597=CARTESIAN_POINT('Ctrl Pts',(0.796153444118959,1.33188468517318,0.605884303066698));
#14598=CARTESIAN_POINT('Ctrl Pts',(0.832065554235658,1.30632915724249,0.555538485325664));
#14599=CARTESIAN_POINT('Ctrl Pts',(0.850258932191534,1.3,0.527308329855003));
#14600=CARTESIAN_POINT('Ctrl Pts',(0.881791875377343,1.3,0.472691670144998));
#14601=CARTESIAN_POINT('Ctrl Pts',(0.897143218189782,1.30632915724249,0.442820664919227));
#14602=CARTESIAN_POINT('Ctrl Pts',(0.92278792026947,1.33188468517318,0.386546956384144));
#14603=CARTESIAN_POINT('Ctrl Pts',(0.933155485613026,1.35110381617461,0.360174810895352));
#14604=CARTESIAN_POINT('Ctrl Pts',(0.948394987258249,1.39534588636318,0.31788699900678));
#14605=CARTESIAN_POINT('Ctrl Pts',(0.954308486908894,1.42336732874239,0.299111603474268));
#14606=CARTESIAN_POINT('Ctrl Pts',(0.961833761492987,1.48491957299738,0.273949373987484));
#14607=CARTESIAN_POINT('Ctrl Pts',(0.963525491562421,1.5184626473304,0.267616567329818));
#14608=CARTESIAN_POINT('Ctrl Pts',(0.963525491562421,1.55,0.267616567329818));
#14609=CARTESIAN_POINT('Origin',(0.,1.55,0.));
#14610=CARTESIAN_POINT('',(-0.713525491562421,1.55,-0.700629269222037));
#14611=CARTESIAN_POINT('Ctrl Pts',(-0.713525491562421,1.55,-0.700629269222037));
#14612=CARTESIAN_POINT('Ctrl Pts',(-0.713525491562421,1.5184626473304,-0.700629269222037));
#14613=CARTESIAN_POINT('Ctrl Pts',(-0.718163997970498,1.48491957299737,
-0.695997784676728));
#14614=CARTESIAN_POINT('Ctrl Pts',(-0.73619249062986,1.42336732874239,-0.676899590973058));
#14615=CARTESIAN_POINT('Ctrl Pts',(-0.749495710301794,1.39534588636318,
-0.662390652284073));
#14616=CARTESIAN_POINT('Ctrl Pts',(-0.778498278845144,1.35110381617461,
-0.62804895077401));
#14617=CARTESIAN_POINT('Ctrl Pts',(-0.796153444118959,1.33188468517318,
-0.605884303066698));
#14618=CARTESIAN_POINT('Ctrl Pts',(-0.832065554235658,1.30632915724249,
-0.555538485325664));
#14619=CARTESIAN_POINT('Ctrl Pts',(-0.850258932191534,1.3,-0.527308329855003));
#14620=CARTESIAN_POINT('Ctrl Pts',(-0.881791875377343,1.3,-0.472691670144998));
#14621=CARTESIAN_POINT('Ctrl Pts',(-0.897143218189782,1.30632915724249,
-0.442820664919227));
#14622=CARTESIAN_POINT('Ctrl Pts',(-0.92278792026947,1.33188468517318,-0.386546956384144));
#14623=CARTESIAN_POINT('Ctrl Pts',(-0.933155485613026,1.35110381617461,
-0.360174810895352));
#14624=CARTESIAN_POINT('Ctrl Pts',(-0.948394987258249,1.39534588636318,
-0.31788699900678));
#14625=CARTESIAN_POINT('Ctrl Pts',(-0.954308486908894,1.42336732874239,
-0.299111603474268));
#14626=CARTESIAN_POINT('Ctrl Pts',(-0.961833761492986,1.48491957299737,
-0.273949373987484));
#14627=CARTESIAN_POINT('Ctrl Pts',(-0.963525491562421,1.5184626473304,-0.267616567329818));
#14628=CARTESIAN_POINT('Ctrl Pts',(-0.963525491562421,1.5815373526696,-0.267616567329818));
#14629=CARTESIAN_POINT('Ctrl Pts',(-0.961833761492986,1.61508042700263,
-0.273949373987484));
#14630=CARTESIAN_POINT('Ctrl Pts',(-0.954308486908894,1.67663267125761,
-0.299111603474268));
#14631=CARTESIAN_POINT('Ctrl Pts',(-0.948394987258249,1.70465411363682,
-0.31788699900678));
#14632=CARTESIAN_POINT('Ctrl Pts',(-0.933155485613026,1.74889618382539,
-0.360174810895352));
#14633=CARTESIAN_POINT('Ctrl Pts',(-0.92278792026947,1.76811531482682,-0.386546956384144));
#14634=CARTESIAN_POINT('Ctrl Pts',(-0.897143218189782,1.79367084275751,
-0.442820664919227));
#14635=CARTESIAN_POINT('Ctrl Pts',(-0.881791875377343,1.8,-0.472691670144998));
#14636=CARTESIAN_POINT('Ctrl Pts',(-0.850258932191534,1.8,-0.527308329855003));
#14637=CARTESIAN_POINT('Ctrl Pts',(-0.832065554235658,1.79367084275751,
-0.555538485325664));
#14638=CARTESIAN_POINT('Ctrl Pts',(-0.796153444118959,1.76811531482682,
-0.605884303066698));
#14639=CARTESIAN_POINT('Ctrl Pts',(-0.778498278845144,1.74889618382539,
-0.62804895077401));
#14640=CARTESIAN_POINT('Ctrl Pts',(-0.749495710301794,1.70465411363682,
-0.662390652284073));
#14641=CARTESIAN_POINT('Ctrl Pts',(-0.73619249062986,1.67663267125761,-0.676899590973058));
#14642=CARTESIAN_POINT('Ctrl Pts',(-0.718163997970498,1.61508042700263,
-0.695997784676728));
#14643=CARTESIAN_POINT('Ctrl Pts',(-0.713525491562421,1.5815373526696,-0.700629269222037));
#14644=CARTESIAN_POINT('Ctrl Pts',(-0.713525491562421,1.55,-0.700629269222037));
#14645=CARTESIAN_POINT('',(-1.28744468918255,1.55,-1.03198167246111));
#14646=CARTESIAN_POINT('',(0.125,1.55,-0.21650635094611));
#14647=CARTESIAN_POINT('',(-1.42894191624432,1.3,-0.825000000000001));
#14648=CARTESIAN_POINT('Ctrl Pts',(-1.42894191624432,1.3,-0.825000000000001));
#14649=CARTESIAN_POINT('Ctrl Pts',(-1.4132207435299,1.3,-0.852229869895949));
#14650=CARTESIAN_POINT('Ctrl Pts',(-1.39561049050871,1.30629366210296,-0.880751161609749));
#14651=CARTESIAN_POINT('Ctrl Pts',(-1.36172049302549,1.33182222741682,-0.932292094146256));
#14652=CARTESIAN_POINT('Ctrl Pts',(-1.34548213209931,1.35105447038507,-0.955340251466735));
#14653=CARTESIAN_POINT('Ctrl Pts',(-1.31917543061769,1.39539254159618,-0.991349264982991));
#14654=CARTESIAN_POINT('Ctrl Pts',(-1.30734972067592,1.42347183818157,-1.00672880483252));
#14655=CARTESIAN_POINT('Ctrl Pts',(-1.29146042158868,1.48505200040818,-1.02703269653942));
#14656=CARTESIAN_POINT('Ctrl Pts',(-1.28744468918255,1.51855708359447,-1.03198167246111));
#14657=CARTESIAN_POINT('Ctrl Pts',(-1.28744468918255,1.55,-1.03198167246111));
#14658=CARTESIAN_POINT('',(-1.42894191624432,1.8,-0.825000000000001));
#14659=CARTESIAN_POINT('Ctrl Pts',(-1.42894191624432,1.8,-0.825000000000001));
#14660=CARTESIAN_POINT('Ctrl Pts',(-1.44466308895875,1.8,-0.797770130104052));
#14661=CARTESIAN_POINT('Ctrl Pts',(-1.46055812562105,1.79370633789704,-0.768258557763732));
#14662=CARTESIAN_POINT('Ctrl Pts',(-1.48824888379079,1.76817777258318,-0.713138492740816));
#14663=CARTESIAN_POINT('Ctrl Pts',(-1.50008999307766,1.74894552961493,-0.687551581002689));
#14664=CARTESIAN_POINT('Ctrl Pts',(-1.51812136280714,1.70460745840382,-0.646764802471699));
#14665=CARTESIAN_POINT('Ctrl Pts',(-1.52552758004446,1.67652816181843,-0.628833667319578));
#14666=CARTESIAN_POINT('Ctrl Pts',(-1.53516661651472,1.61494799959182,-0.60492118480825));
#14667=CARTESIAN_POINT('Ctrl Pts',(-1.53744468918255,1.58144291640553,-0.598968970568896));
#14668=CARTESIAN_POINT('Ctrl Pts',(-1.53744468918255,1.51855708359447,-0.598968970568896));
#14669=CARTESIAN_POINT('Ctrl Pts',(-1.53516661651472,1.48505200040818,-0.60492118480825));
#14670=CARTESIAN_POINT('Ctrl Pts',(-1.52552758004446,1.42347183818157,-0.628833667319578));
#14671=CARTESIAN_POINT('Ctrl Pts',(-1.51812136280714,1.39539254159618,-0.646764802471699));
#14672=CARTESIAN_POINT('Ctrl Pts',(-1.50008999307766,1.35105447038507,-0.687551581002689));
#14673=CARTESIAN_POINT('Ctrl Pts',(-1.48824888379079,1.33182222741682,-0.713138492740816));
#14674=CARTESIAN_POINT('Ctrl Pts',(-1.46055812562105,1.30629366210296,-0.768258557763732));
#14675=CARTESIAN_POINT('Ctrl Pts',(-1.44466308895875,1.3,-0.797770130104052));
#14676=CARTESIAN_POINT('Ctrl Pts',(-1.42894191624432,1.3,-0.825000000000001));
#14677=CARTESIAN_POINT('Ctrl Pts',(-1.28744468918255,1.55,-1.03198167246111));
#14678=CARTESIAN_POINT('Ctrl Pts',(-1.28744468918255,1.58144291640553,-1.03198167246111));
#14679=CARTESIAN_POINT('Ctrl Pts',(-1.29146042158868,1.61494799959182,-1.02703269653942));
#14680=CARTESIAN_POINT('Ctrl Pts',(-1.30734972067592,1.67652816181843,-1.00672880483252));
#14681=CARTESIAN_POINT('Ctrl Pts',(-1.31917543061769,1.70460745840382,-0.991349264982991));
#14682=CARTESIAN_POINT('Ctrl Pts',(-1.34548213209931,1.74894552961493,-0.955340251466734));
#14683=CARTESIAN_POINT('Ctrl Pts',(-1.36172049302549,1.76817777258318,-0.932292094146256));
#14684=CARTESIAN_POINT('Ctrl Pts',(-1.39561049050871,1.79370633789704,-0.880751161609749));
#14685=CARTESIAN_POINT('Ctrl Pts',(-1.4132207435299,1.8,-0.852229869895949));
#14686=CARTESIAN_POINT('Ctrl Pts',(-1.42894191624432,1.8,-0.825000000000001));
#14687=CARTESIAN_POINT('Origin',(0.,1.55,0.));
#14688=CARTESIAN_POINT('',(-1.65,0.85,-2.02066721859313E-16));
#14689=CARTESIAN_POINT('Origin',(0.,0.85,0.));
#14690=CARTESIAN_POINT('',(-1.65,2.25,-2.02066721859313E-16));
#14691=CARTESIAN_POINT('',(-1.65,1.55,-2.02066721859313E-16));
#14692=CARTESIAN_POINT('Origin',(0.,2.25,0.));
#14693=CARTESIAN_POINT('',(-1.42894191624432,1.3,0.825));
#14694=CARTESIAN_POINT('',(-1.42894191624432,1.8,0.825));
#14695=CARTESIAN_POINT('Ctrl Pts',(-1.42894191624432,1.3,0.825));
#14696=CARTESIAN_POINT('Ctrl Pts',(-1.44466308895875,1.3,0.797770130104051));
#14697=CARTESIAN_POINT('Ctrl Pts',(-1.46055812562105,1.30629366210296,0.768258557763731));
#14698=CARTESIAN_POINT('Ctrl Pts',(-1.48824888379079,1.33182222741682,0.713138492740815));
#14699=CARTESIAN_POINT('Ctrl Pts',(-1.50008999307766,1.35105447038507,0.687551581002688));
#14700=CARTESIAN_POINT('Ctrl Pts',(-1.51812136280714,1.39539254159618,0.646764802471698));
#14701=CARTESIAN_POINT('Ctrl Pts',(-1.52552758004446,1.42347183818157,0.628833667319577));
#14702=CARTESIAN_POINT('Ctrl Pts',(-1.53516661651472,1.48505200040818,0.604921184808249));
#14703=CARTESIAN_POINT('Ctrl Pts',(-1.53744468918255,1.51855708359447,0.598968970568895));
#14704=CARTESIAN_POINT('Ctrl Pts',(-1.53744468918255,1.58144291640553,0.598968970568895));
#14705=CARTESIAN_POINT('Ctrl Pts',(-1.53516661651472,1.61494799959182,0.604921184808249));
#14706=CARTESIAN_POINT('Ctrl Pts',(-1.52552758004446,1.67652816181843,0.628833667319577));
#14707=CARTESIAN_POINT('Ctrl Pts',(-1.51812136280714,1.70460745840382,0.646764802471698));
#14708=CARTESIAN_POINT('Ctrl Pts',(-1.50008999307766,1.74894552961493,0.687551581002688));
#14709=CARTESIAN_POINT('Ctrl Pts',(-1.48824888379079,1.76817777258318,0.713138492740815));
#14710=CARTESIAN_POINT('Ctrl Pts',(-1.46055812562105,1.79370633789704,0.768258557763731));
#14711=CARTESIAN_POINT('Ctrl Pts',(-1.44466308895875,1.8,0.797770130104051));
#14712=CARTESIAN_POINT('Ctrl Pts',(-1.42894191624432,1.8,0.825));
#14713=CARTESIAN_POINT('',(-1.28744468918255,1.55,1.03198167246111));
#14714=CARTESIAN_POINT('Ctrl Pts',(-1.42894191624432,1.8,0.825));
#14715=CARTESIAN_POINT('Ctrl Pts',(-1.4132207435299,1.8,0.852229869895948));
#14716=CARTESIAN_POINT('Ctrl Pts',(-1.39561049050871,1.79370633789704,0.880751161609747));
#14717=CARTESIAN_POINT('Ctrl Pts',(-1.36172049302549,1.76817777258318,0.932292094146255));
#14718=CARTESIAN_POINT('Ctrl Pts',(-1.34548213209931,1.74894552961493,0.955340251466733));
#14719=CARTESIAN_POINT('Ctrl Pts',(-1.31917543061769,1.70460745840382,0.991349264982989));
#14720=CARTESIAN_POINT('Ctrl Pts',(-1.30734972067592,1.67652816181843,1.00672880483252));
#14721=CARTESIAN_POINT('Ctrl Pts',(-1.29146042158868,1.61494799959182,1.02703269653942));
#14722=CARTESIAN_POINT('Ctrl Pts',(-1.28744468918255,1.58144291640553,1.03198167246111));
#14723=CARTESIAN_POINT('Ctrl Pts',(-1.28744468918255,1.55,1.03198167246111));
#14724=CARTESIAN_POINT('Ctrl Pts',(-1.28744468918255,1.55,1.03198167246111));
#14725=CARTESIAN_POINT('Ctrl Pts',(-1.28744468918255,1.51855708359447,1.03198167246111));
#14726=CARTESIAN_POINT('Ctrl Pts',(-1.29146042158868,1.48505200040818,1.02703269653942));
#14727=CARTESIAN_POINT('Ctrl Pts',(-1.30734972067592,1.42347183818157,1.00672880483252));
#14728=CARTESIAN_POINT('Ctrl Pts',(-1.31917543061769,1.39539254159618,0.99134926498299));
#14729=CARTESIAN_POINT('Ctrl Pts',(-1.34548213209931,1.35105447038508,0.955340251466733));
#14730=CARTESIAN_POINT('Ctrl Pts',(-1.36172049302549,1.33182222741682,0.932292094146255));
#14731=CARTESIAN_POINT('Ctrl Pts',(-1.39561049050871,1.30629366210296,0.880751161609748));
#14732=CARTESIAN_POINT('Ctrl Pts',(-1.4132207435299,1.3,0.852229869895949));
#14733=CARTESIAN_POINT('Ctrl Pts',(-1.42894191624432,1.3,0.825));
#14734=CARTESIAN_POINT('',(1.42894191624432,1.8,-0.825));
#14735=CARTESIAN_POINT('',(1.42894191624432,1.3,-0.825));
#14736=CARTESIAN_POINT('Ctrl Pts',(1.42894191624432,1.8,-0.825));
#14737=CARTESIAN_POINT('Ctrl Pts',(1.4132207435299,1.8,-0.852229869895949));
#14738=CARTESIAN_POINT('Ctrl Pts',(1.39561049050871,1.79370633789704,-0.880751161609748));
#14739=CARTESIAN_POINT('Ctrl Pts',(1.36172049302549,1.76817777258318,-0.932292094146255));
#14740=CARTESIAN_POINT('Ctrl Pts',(1.34548213209931,1.74894552961493,-0.955340251466734));
#14741=CARTESIAN_POINT('Ctrl Pts',(1.31917543061769,1.70460745840382,-0.99134926498299));
#14742=CARTESIAN_POINT('Ctrl Pts',(1.30734972067592,1.67652816181843,-1.00672880483252));
#14743=CARTESIAN_POINT('Ctrl Pts',(1.29146042158868,1.61494799959182,-1.02703269653942));
#14744=CARTESIAN_POINT('Ctrl Pts',(1.28744468918255,1.58144291640553,-1.03198167246111));
#14745=CARTESIAN_POINT('Ctrl Pts',(1.28744468918255,1.51855708359447,-1.03198167246111));
#14746=CARTESIAN_POINT('Ctrl Pts',(1.29146042158868,1.48505200040818,-1.02703269653942));
#14747=CARTESIAN_POINT('Ctrl Pts',(1.30734972067592,1.42347183818157,-1.00672880483252));
#14748=CARTESIAN_POINT('Ctrl Pts',(1.31917543061769,1.39539254159618,-0.99134926498299));
#14749=CARTESIAN_POINT('Ctrl Pts',(1.34548213209931,1.35105447038507,-0.955340251466734));
#14750=CARTESIAN_POINT('Ctrl Pts',(1.36172049302549,1.33182222741682,-0.932292094146255));
#14751=CARTESIAN_POINT('Ctrl Pts',(1.39561049050871,1.30629366210296,-0.880751161609748));
#14752=CARTESIAN_POINT('Ctrl Pts',(1.4132207435299,1.3,-0.852229869895948));
#14753=CARTESIAN_POINT('Ctrl Pts',(1.42894191624432,1.3,-0.825));
#14754=CARTESIAN_POINT('',(1.53744468918255,1.55,-0.598968970568895));
#14755=CARTESIAN_POINT('Ctrl Pts',(1.42894191624432,1.3,-0.825));
#14756=CARTESIAN_POINT('Ctrl Pts',(1.44466308895875,1.3,-0.797770130104051));
#14757=CARTESIAN_POINT('Ctrl Pts',(1.46055812562105,1.30629366210296,-0.768258557763731));
#14758=CARTESIAN_POINT('Ctrl Pts',(1.48824888379079,1.33182222741682,-0.713138492740815));
#14759=CARTESIAN_POINT('Ctrl Pts',(1.50008999307766,1.35105447038507,-0.687551581002688));
#14760=CARTESIAN_POINT('Ctrl Pts',(1.51812136280714,1.39539254159618,-0.646764802471698));
#14761=CARTESIAN_POINT('Ctrl Pts',(1.52552758004446,1.42347183818157,-0.628833667319577));
#14762=CARTESIAN_POINT('Ctrl Pts',(1.53516661651472,1.48505200040818,-0.604921184808249));
#14763=CARTESIAN_POINT('Ctrl Pts',(1.53744468918255,1.51855708359447,-0.598968970568895));
#14764=CARTESIAN_POINT('Ctrl Pts',(1.53744468918255,1.55,-0.598968970568895));
#14765=CARTESIAN_POINT('Ctrl Pts',(1.53744468918255,1.55,-0.598968970568895));
#14766=CARTESIAN_POINT('Ctrl Pts',(1.53744468918255,1.58144291640553,-0.598968970568895));
#14767=CARTESIAN_POINT('Ctrl Pts',(1.53516661651472,1.61494799959182,-0.604921184808249));
#14768=CARTESIAN_POINT('Ctrl Pts',(1.52552758004446,1.67652816181843,-0.628833667319577));
#14769=CARTESIAN_POINT('Ctrl Pts',(1.51812136280714,1.70460745840382,-0.646764802471698));
#14770=CARTESIAN_POINT('Ctrl Pts',(1.50008999307766,1.74894552961493,-0.687551581002688));
#14771=CARTESIAN_POINT('Ctrl Pts',(1.48824888379079,1.76817777258318,-0.713138492740815));
#14772=CARTESIAN_POINT('Ctrl Pts',(1.46055812562105,1.79370633789704,-0.768258557763731));
#14773=CARTESIAN_POINT('Ctrl Pts',(1.44466308895875,1.8,-0.797770130104051));
#14774=CARTESIAN_POINT('Ctrl Pts',(1.42894191624432,1.8,-0.825));
#14775=CARTESIAN_POINT('',(0.,1.3,-1.65));
#14776=CARTESIAN_POINT('',(0.,1.8,-1.65));
#14777=CARTESIAN_POINT('Ctrl Pts',(1.38777878078145E-17,1.3,-1.65));
#14778=CARTESIAN_POINT('Ctrl Pts',(0.0314423454288489,1.3,-1.65));
#14779=CARTESIAN_POINT('Ctrl Pts',(0.0649476351123396,1.30629366210296,
-1.64900971937348));
#14780=CARTESIAN_POINT('Ctrl Pts',(0.126528390765307,1.33182222741682,-1.64543058688707));
#14781=CARTESIAN_POINT('Ctrl Pts',(0.154607860978348,1.35105447038507,-1.64289183246942));
#14782=CARTESIAN_POINT('Ctrl Pts',(0.198945932189457,1.39539254159618,-1.63811406745469));
#14783=CARTESIAN_POINT('Ctrl Pts',(0.218177859368546,1.42347183818157,-1.63556247215209));
#14784=CARTESIAN_POINT('Ctrl Pts',(0.243706194926033,1.48505200040818,-1.63195388134767));
#14785=CARTESIAN_POINT('Ctrl Pts',(0.25,1.51855708359447,-1.63095064303001));
#14786=CARTESIAN_POINT('Ctrl Pts',(0.25,1.58144291640553,-1.63095064303001));
#14787=CARTESIAN_POINT('Ctrl Pts',(0.243706194926033,1.61494799959182,-1.63195388134767));
#14788=CARTESIAN_POINT('Ctrl Pts',(0.218177859368546,1.67652816181843,-1.63556247215209));
#14789=CARTESIAN_POINT('Ctrl Pts',(0.198945932189457,1.70460745840382,-1.63811406745469));
#14790=CARTESIAN_POINT('Ctrl Pts',(0.154607860978349,1.74894552961493,-1.64289183246942));
#14791=CARTESIAN_POINT('Ctrl Pts',(0.126528390765307,1.76817777258318,-1.64543058688707));
#14792=CARTESIAN_POINT('Ctrl Pts',(0.0649476351123398,1.79370633789704,
-1.64900971937348));
#14793=CARTESIAN_POINT('Ctrl Pts',(0.031442345428849,1.8,-1.65));
#14794=CARTESIAN_POINT('Ctrl Pts',(7.63278329429795E-17,1.8,-1.65));
#14795=CARTESIAN_POINT('',(-0.25,1.55,-1.63095064303001));
#14796=CARTESIAN_POINT('Ctrl Pts',(9.0205620750794E-17,1.8,-1.65));
#14797=CARTESIAN_POINT('Ctrl Pts',(-0.0314423454288488,1.8,-1.65));
#14798=CARTESIAN_POINT('Ctrl Pts',(-0.0649476351123396,1.79370633789704,
-1.64900971937348));
#14799=CARTESIAN_POINT('Ctrl Pts',(-0.126528390765307,1.76817777258318,
-1.64543058688707));
#14800=CARTESIAN_POINT('Ctrl Pts',(-0.154607860978348,1.74894552961493,
-1.64289183246942));
#14801=CARTESIAN_POINT('Ctrl Pts',(-0.198945932189456,1.70460745840382,
-1.63811406745469));
#14802=CARTESIAN_POINT('Ctrl Pts',(-0.218177859368546,1.67652816181843,
-1.63556247215209));
#14803=CARTESIAN_POINT('Ctrl Pts',(-0.243706194926033,1.61494799959182,
-1.63195388134767));
#14804=CARTESIAN_POINT('Ctrl Pts',(-0.25,1.58144291640553,-1.63095064303001));
#14805=CARTESIAN_POINT('Ctrl Pts',(-0.25,1.55,-1.63095064303001));
#14806=CARTESIAN_POINT('Ctrl Pts',(-0.25,1.55,-1.63095064303001));
#14807=CARTESIAN_POINT('Ctrl Pts',(-0.25,1.51855708359447,-1.63095064303001));
#14808=CARTESIAN_POINT('Ctrl Pts',(-0.243706194926033,1.48505200040818,
-1.63195388134767));
#14809=CARTESIAN_POINT('Ctrl Pts',(-0.218177859368546,1.42347183818157,
-1.63556247215209));
#14810=CARTESIAN_POINT('Ctrl Pts',(-0.198945932189457,1.39539254159618,
-1.63811406745469));
#14811=CARTESIAN_POINT('Ctrl Pts',(-0.154607860978349,1.35105447038507,
-1.64289183246942));
#14812=CARTESIAN_POINT('Ctrl Pts',(-0.126528390765307,1.33182222741682,
-1.64543058688707));
#14813=CARTESIAN_POINT('Ctrl Pts',(-0.0649476351123398,1.30629366210296,
-1.64900971937348));
#14814=CARTESIAN_POINT('Ctrl Pts',(-0.031442345428849,1.3,-1.65));
#14815=CARTESIAN_POINT('Ctrl Pts',(-4.85722573273506E-17,1.3,-1.65));
#14816=CARTESIAN_POINT('',(0.,1.8,1.65));
#14817=CARTESIAN_POINT('',(0.,1.3,1.65));
#14818=CARTESIAN_POINT('Ctrl Pts',(8.32667268468867E-17,1.8,1.65));
#14819=CARTESIAN_POINT('Ctrl Pts',(0.031442345428849,1.8,1.65));
#14820=CARTESIAN_POINT('Ctrl Pts',(0.0649476351123398,1.79370633789704,
1.64900971937348));
#14821=CARTESIAN_POINT('Ctrl Pts',(0.126528390765307,1.76817777258318,1.64543058688707));
#14822=CARTESIAN_POINT('Ctrl Pts',(0.154607860978349,1.74894552961493,1.64289183246942));
#14823=CARTESIAN_POINT('Ctrl Pts',(0.198945932189457,1.70460745840382,1.63811406745469));
#14824=CARTESIAN_POINT('Ctrl Pts',(0.218177859368546,1.67652816181843,1.63556247215209));
#14825=CARTESIAN_POINT('Ctrl Pts',(0.243706194926033,1.61494799959182,1.63195388134767));
#14826=CARTESIAN_POINT('Ctrl Pts',(0.25,1.58144291640553,1.63095064303001));
#14827=CARTESIAN_POINT('Ctrl Pts',(0.25,1.51855708359447,1.63095064303001));
#14828=CARTESIAN_POINT('Ctrl Pts',(0.243706194926033,1.48505200040818,1.63195388134767));
#14829=CARTESIAN_POINT('Ctrl Pts',(0.218177859368546,1.42347183818157,1.63556247215209));
#14830=CARTESIAN_POINT('Ctrl Pts',(0.198945932189457,1.39539254159618,1.63811406745469));
#14831=CARTESIAN_POINT('Ctrl Pts',(0.154607860978348,1.35105447038507,1.64289183246942));
#14832=CARTESIAN_POINT('Ctrl Pts',(0.126528390765307,1.33182222741682,1.64543058688707));
#14833=CARTESIAN_POINT('Ctrl Pts',(0.0649476351123397,1.30629366210296,
1.64900971937348));
#14834=CARTESIAN_POINT('Ctrl Pts',(0.0314423454288488,1.3,1.65));
#14835=CARTESIAN_POINT('Ctrl Pts',(-1.38777878078145E-17,1.3,1.65));
#14836=CARTESIAN_POINT('',(-0.25,1.55,1.63095064303001));
#14837=CARTESIAN_POINT('Ctrl Pts',(-5.55111512312578E-17,1.3,1.65));
#14838=CARTESIAN_POINT('Ctrl Pts',(-0.031442345428849,1.3,1.65));
#14839=CARTESIAN_POINT('Ctrl Pts',(-0.0649476351123398,1.30629366210296,
1.64900971937348));
#14840=CARTESIAN_POINT('Ctrl Pts',(-0.126528390765307,1.33182222741682,
1.64543058688707));
#14841=CARTESIAN_POINT('Ctrl Pts',(-0.154607860978349,1.35105447038507,
1.64289183246942));
#14842=CARTESIAN_POINT('Ctrl Pts',(-0.198945932189457,1.39539254159618,
1.63811406745469));
#14843=CARTESIAN_POINT('Ctrl Pts',(-0.218177859368546,1.42347183818157,
1.63556247215209));
#14844=CARTESIAN_POINT('Ctrl Pts',(-0.243706194926033,1.48505200040818,
1.63195388134767));
#14845=CARTESIAN_POINT('Ctrl Pts',(-0.25,1.51855708359447,1.63095064303001));
#14846=CARTESIAN_POINT('Ctrl Pts',(-0.25,1.55,1.63095064303001));
#14847=CARTESIAN_POINT('Ctrl Pts',(-0.25,1.55,1.63095064303001));
#14848=CARTESIAN_POINT('Ctrl Pts',(-0.25,1.58144291640553,1.63095064303001));
#14849=CARTESIAN_POINT('Ctrl Pts',(-0.243706194926033,1.61494799959182,
1.63195388134767));
#14850=CARTESIAN_POINT('Ctrl Pts',(-0.218177859368546,1.67652816181843,
1.63556247215209));
#14851=CARTESIAN_POINT('Ctrl Pts',(-0.198945932189456,1.70460745840382,
1.63811406745469));
#14852=CARTESIAN_POINT('Ctrl Pts',(-0.154607860978348,1.74894552961493,
1.64289183246942));
#14853=CARTESIAN_POINT('Ctrl Pts',(-0.126528390765307,1.76817777258318,
1.64543058688707));
#14854=CARTESIAN_POINT('Ctrl Pts',(-0.0649476351123396,1.79370633789704,
1.64900971937348));
#14855=CARTESIAN_POINT('Ctrl Pts',(-0.0314423454288488,1.8,1.65));
#14856=CARTESIAN_POINT('Ctrl Pts',(7.63278329429795E-17,1.8,1.65));
#14857=CARTESIAN_POINT('Origin',(0.,1.55,0.));
#14858=CARTESIAN_POINT('',(-0.713525491562421,1.55,0.700629269222037));
#14859=CARTESIAN_POINT('',(0.125,1.55,0.21650635094611));
#14860=CARTESIAN_POINT('Ctrl Pts',(-0.713525491562421,1.55,0.700629269222037));
#14861=CARTESIAN_POINT('Ctrl Pts',(-0.713525491562421,1.5815373526696,0.700629269222037));
#14862=CARTESIAN_POINT('Ctrl Pts',(-0.718163997970498,1.61508042700263,
0.695997784676727));
#14863=CARTESIAN_POINT('Ctrl Pts',(-0.73619249062986,1.67663267125761,0.676899590973058));
#14864=CARTESIAN_POINT('Ctrl Pts',(-0.749495710301795,1.70465411363682,
0.662390652284073));
#14865=CARTESIAN_POINT('Ctrl Pts',(-0.778498278845144,1.74889618382539,
0.628048950774009));
#14866=CARTESIAN_POINT('Ctrl Pts',(-0.796153444118959,1.76811531482682,
0.605884303066698));
#14867=CARTESIAN_POINT('Ctrl Pts',(-0.832065554235658,1.79367084275751,
0.555538485325663));
#14868=CARTESIAN_POINT('Ctrl Pts',(-0.850258932191534,1.8,0.527308329855002));
#14869=CARTESIAN_POINT('Ctrl Pts',(-0.881791875377343,1.8,0.472691670144998));
#14870=CARTESIAN_POINT('Ctrl Pts',(-0.897143218189782,1.79367084275751,
0.442820664919227));
#14871=CARTESIAN_POINT('Ctrl Pts',(-0.92278792026947,1.76811531482682,0.386546956384144));
#14872=CARTESIAN_POINT('Ctrl Pts',(-0.933155485613026,1.74889618382539,
0.360174810895352));
#14873=CARTESIAN_POINT('Ctrl Pts',(-0.948394987258249,1.70465411363682,
0.31788699900678));
#14874=CARTESIAN_POINT('Ctrl Pts',(-0.954308486908894,1.67663267125761,
0.299111603474267));
#14875=CARTESIAN_POINT('Ctrl Pts',(-0.961833761492987,1.61508042700263,
0.273949373987484));
#14876=CARTESIAN_POINT('Ctrl Pts',(-0.963525491562421,1.5815373526696,0.267616567329817));
#14877=CARTESIAN_POINT('Ctrl Pts',(-0.963525491562421,1.5184626473304,0.267616567329817));
#14878=CARTESIAN_POINT('Ctrl Pts',(-0.961833761492987,1.48491957299737,
0.273949373987484));
#14879=CARTESIAN_POINT('Ctrl Pts',(-0.954308486908894,1.42336732874239,
0.299111603474267));
#14880=CARTESIAN_POINT('Ctrl Pts',(-0.948394987258249,1.39534588636318,
0.31788699900678));
#14881=CARTESIAN_POINT('Ctrl Pts',(-0.933155485613026,1.35110381617461,
0.360174810895352));
#14882=CARTESIAN_POINT('Ctrl Pts',(-0.92278792026947,1.33188468517318,0.386546956384144));
#14883=CARTESIAN_POINT('Ctrl Pts',(-0.897143218189782,1.30632915724249,
0.442820664919227));
#14884=CARTESIAN_POINT('Ctrl Pts',(-0.881791875377343,1.3,0.472691670144998));
#14885=CARTESIAN_POINT('Ctrl Pts',(-0.850258932191534,1.3,0.527308329855002));
#14886=CARTESIAN_POINT('Ctrl Pts',(-0.832065554235658,1.30632915724249,
0.555538485325663));
#14887=CARTESIAN_POINT('Ctrl Pts',(-0.796153444118959,1.33188468517318,
0.605884303066698));
#14888=CARTESIAN_POINT('Ctrl Pts',(-0.778498278845144,1.35110381617461,
0.628048950774009));
#14889=CARTESIAN_POINT('Ctrl Pts',(-0.749495710301795,1.39534588636318,
0.662390652284073));
#14890=CARTESIAN_POINT('Ctrl Pts',(-0.73619249062986,1.42336732874239,0.676899590973058));
#14891=CARTESIAN_POINT('Ctrl Pts',(-0.718163997970498,1.48491957299737,
0.695997784676727));
#14892=CARTESIAN_POINT('Ctrl Pts',(-0.713525491562421,1.5184626473304,0.700629269222037));
#14893=CARTESIAN_POINT('Ctrl Pts',(-0.713525491562421,1.55,0.700629269222037));
#14894=CARTESIAN_POINT('Origin',(0.,1.55,0.));
#14895=CARTESIAN_POINT('',(0.963525491562421,1.55,-0.267616567329817));
#14896=CARTESIAN_POINT('Ctrl Pts',(0.963525491562421,1.55,-0.267616567329817));
#14897=CARTESIAN_POINT('Ctrl Pts',(0.963525491562421,1.5184626473304,-0.267616567329817));
#14898=CARTESIAN_POINT('Ctrl Pts',(0.961833761492987,1.48491957299737,-0.273949373987484));
#14899=CARTESIAN_POINT('Ctrl Pts',(0.954308486908894,1.42336732874239,-0.299111603474267));
#14900=CARTESIAN_POINT('Ctrl Pts',(0.948394987258249,1.39534588636318,-0.31788699900678));
#14901=CARTESIAN_POINT('Ctrl Pts',(0.933155485613026,1.35110381617461,-0.360174810895352));
#14902=CARTESIAN_POINT('Ctrl Pts',(0.92278792026947,1.33188468517318,-0.386546956384144));
#14903=CARTESIAN_POINT('Ctrl Pts',(0.897143218189782,1.30632915724249,-0.442820664919227));
#14904=CARTESIAN_POINT('Ctrl Pts',(0.881791875377343,1.3,-0.472691670144998));
#14905=CARTESIAN_POINT('Ctrl Pts',(0.850258932191534,1.3,-0.527308329855002));
#14906=CARTESIAN_POINT('Ctrl Pts',(0.832065554235658,1.30632915724249,-0.555538485325663));
#14907=CARTESIAN_POINT('Ctrl Pts',(0.796153444118959,1.33188468517318,-0.605884303066698));
#14908=CARTESIAN_POINT('Ctrl Pts',(0.778498278845144,1.35110381617461,-0.628048950774009));
#14909=CARTESIAN_POINT('Ctrl Pts',(0.749495710301795,1.39534588636318,-0.662390652284073));
#14910=CARTESIAN_POINT('Ctrl Pts',(0.73619249062986,1.42336732874239,-0.676899590973058));
#14911=CARTESIAN_POINT('Ctrl Pts',(0.718163997970498,1.48491957299737,-0.695997784676727));
#14912=CARTESIAN_POINT('Ctrl Pts',(0.713525491562421,1.5184626473304,-0.700629269222037));
#14913=CARTESIAN_POINT('Ctrl Pts',(0.713525491562421,1.5815373526696,-0.700629269222037));
#14914=CARTESIAN_POINT('Ctrl Pts',(0.718163997970498,1.61508042700263,-0.695997784676727));
#14915=CARTESIAN_POINT('Ctrl Pts',(0.73619249062986,1.67663267125761,-0.676899590973058));
#14916=CARTESIAN_POINT('Ctrl Pts',(0.749495710301795,1.70465411363682,-0.662390652284073));
#14917=CARTESIAN_POINT('Ctrl Pts',(0.778498278845144,1.74889618382539,-0.628048950774009));
#14918=CARTESIAN_POINT('Ctrl Pts',(0.796153444118959,1.76811531482682,-0.605884303066698));
#14919=CARTESIAN_POINT('Ctrl Pts',(0.832065554235658,1.79367084275751,-0.555538485325663));
#14920=CARTESIAN_POINT('Ctrl Pts',(0.850258932191534,1.8,-0.527308329855002));
#14921=CARTESIAN_POINT('Ctrl Pts',(0.881791875377343,1.8,-0.472691670144998));
#14922=CARTESIAN_POINT('Ctrl Pts',(0.897143218189782,1.79367084275751,-0.442820664919227));
#14923=CARTESIAN_POINT('Ctrl Pts',(0.92278792026947,1.76811531482682,-0.386546956384144));
#14924=CARTESIAN_POINT('Ctrl Pts',(0.933155485613026,1.74889618382539,-0.360174810895352));
#14925=CARTESIAN_POINT('Ctrl Pts',(0.948394987258249,1.70465411363682,-0.31788699900678));
#14926=CARTESIAN_POINT('Ctrl Pts',(0.954308486908894,1.67663267125761,-0.299111603474267));
#14927=CARTESIAN_POINT('Ctrl Pts',(0.961833761492987,1.61508042700263,-0.273949373987484));
#14928=CARTESIAN_POINT('Ctrl Pts',(0.963525491562421,1.5815373526696,-0.267616567329817));
#14929=CARTESIAN_POINT('Ctrl Pts',(0.963525491562421,1.55,-0.267616567329817));
#14930=CARTESIAN_POINT('',(0.125,1.55,0.21650635094611));
#14931=CARTESIAN_POINT('Origin',(0.,1.55,0.));
#14932=CARTESIAN_POINT('',(-0.25,1.55,-0.968245836551854));
#14933=CARTESIAN_POINT('',(-0.25,1.55,0.));
#14934=CARTESIAN_POINT('Ctrl Pts',(-0.25,1.55,-0.968245836551854));
#14935=CARTESIAN_POINT('Ctrl Pts',(-0.25,1.5815373526696,-0.968245836551854));
#14936=CARTESIAN_POINT('Ctrl Pts',(-0.243669763522489,1.61508042700263,
-0.969947158664211));
#14937=CARTESIAN_POINT('Ctrl Pts',(-0.218115996279034,1.67663267125761,
-0.976011194447325));
#14938=CARTESIAN_POINT('Ctrl Pts',(-0.198899276956455,1.70465411363682,
-0.980277651290853));
#14939=CARTESIAN_POINT('Ctrl Pts',(-0.154657206767882,1.74889618382539,
-0.988223761669361));
#14940=CARTESIAN_POINT('Ctrl Pts',(-0.126634476150511,1.76811531482682,
-0.992431259450842));
#14941=CARTESIAN_POINT('Ctrl Pts',(-0.0650776639541238,1.79367084275751,
-0.99835915024489));
#14942=CARTESIAN_POINT('Ctrl Pts',(-0.0315329431858092,1.8,-1.));
#14943=CARTESIAN_POINT('Ctrl Pts',(0.0315329431858092,1.8,-1.));
#14944=CARTESIAN_POINT('Ctrl Pts',(0.0650776639541238,1.79367084275751,
-0.99835915024489));
#14945=CARTESIAN_POINT('Ctrl Pts',(0.126634476150511,1.76811531482682,-0.992431259450842));
#14946=CARTESIAN_POINT('Ctrl Pts',(0.154657206767882,1.74889618382539,-0.988223761669361));
#14947=CARTESIAN_POINT('Ctrl Pts',(0.198899276956455,1.70465411363682,-0.980277651290853));
#14948=CARTESIAN_POINT('Ctrl Pts',(0.218115996279034,1.67663267125761,-0.976011194447325));
#14949=CARTESIAN_POINT('Ctrl Pts',(0.243669763522488,1.61508042700263,-0.969947158664211));
#14950=CARTESIAN_POINT('Ctrl Pts',(0.25,1.5815373526696,-0.968245836551854));
#14951=CARTESIAN_POINT('Ctrl Pts',(0.25,1.5184626473304,-0.968245836551854));
#14952=CARTESIAN_POINT('Ctrl Pts',(0.243669763522488,1.48491957299737,-0.969947158664211));
#14953=CARTESIAN_POINT('Ctrl Pts',(0.218115996279034,1.42336732874239,-0.976011194447325));
#14954=CARTESIAN_POINT('Ctrl Pts',(0.198899276956455,1.39534588636318,-0.980277651290853));
#14955=CARTESIAN_POINT('Ctrl Pts',(0.154657206767882,1.35110381617461,-0.988223761669361));
#14956=CARTESIAN_POINT('Ctrl Pts',(0.126634476150511,1.33188468517318,-0.992431259450842));
#14957=CARTESIAN_POINT('Ctrl Pts',(0.0650776639541239,1.30632915724249,
-0.99835915024489));
#14958=CARTESIAN_POINT('Ctrl Pts',(0.0315329431858092,1.3,-1.));
#14959=CARTESIAN_POINT('Ctrl Pts',(-0.0315329431858092,1.3,-1.));
#14960=CARTESIAN_POINT('Ctrl Pts',(-0.0650776639541239,1.30632915724249,
-0.99835915024489));
#14961=CARTESIAN_POINT('Ctrl Pts',(-0.126634476150511,1.33188468517318,
-0.992431259450842));
#14962=CARTESIAN_POINT('Ctrl Pts',(-0.154657206767882,1.35110381617461,
-0.988223761669361));
#14963=CARTESIAN_POINT('Ctrl Pts',(-0.198899276956455,1.39534588636318,
-0.980277651290853));
#14964=CARTESIAN_POINT('Ctrl Pts',(-0.218115996279034,1.42336732874239,
-0.976011194447325));
#14965=CARTESIAN_POINT('Ctrl Pts',(-0.243669763522489,1.48491957299737,
-0.969947158664211));
#14966=CARTESIAN_POINT('Ctrl Pts',(-0.25,1.5184626473304,-0.968245836551854));
#14967=CARTESIAN_POINT('Ctrl Pts',(-0.25,1.55,-0.968245836551854));
#14968=CARTESIAN_POINT('Origin',(0.,1.55,0.));
#14969=CARTESIAN_POINT('',(-0.25,1.55,0.968245836551854));
#14970=CARTESIAN_POINT('Ctrl Pts',(-0.25,1.55,0.968245836551854));
#14971=CARTESIAN_POINT('Ctrl Pts',(-0.25,1.5184626473304,0.968245836551854));
#14972=CARTESIAN_POINT('Ctrl Pts',(-0.243669763522489,1.48491957299737,
0.969947158664211));
#14973=CARTESIAN_POINT('Ctrl Pts',(-0.218115996279034,1.42336732874239,
0.976011194447325));
#14974=CARTESIAN_POINT('Ctrl Pts',(-0.198899276956455,1.39534588636318,
0.980277651290853));
#14975=CARTESIAN_POINT('Ctrl Pts',(-0.154657206767882,1.35110381617461,
0.988223761669361));
#14976=CARTESIAN_POINT('Ctrl Pts',(-0.126634476150511,1.33188468517318,
0.992431259450842));
#14977=CARTESIAN_POINT('Ctrl Pts',(-0.065077663954124,1.30632915724249,
0.99835915024489));
#14978=CARTESIAN_POINT('Ctrl Pts',(-0.0315329431858092,1.3,1.));
#14979=CARTESIAN_POINT('Ctrl Pts',(0.0315329431858092,1.3,1.));
#14980=CARTESIAN_POINT('Ctrl Pts',(0.065077663954124,1.30632915724249,0.99835915024489));
#14981=CARTESIAN_POINT('Ctrl Pts',(0.126634476150511,1.33188468517318,0.992431259450842));
#14982=CARTESIAN_POINT('Ctrl Pts',(0.154657206767882,1.35110381617461,0.988223761669361));
#14983=CARTESIAN_POINT('Ctrl Pts',(0.198899276956455,1.39534588636318,0.980277651290853));
#14984=CARTESIAN_POINT('Ctrl Pts',(0.218115996279034,1.42336732874239,0.976011194447325));
#14985=CARTESIAN_POINT('Ctrl Pts',(0.243669763522488,1.48491957299737,0.969947158664211));
#14986=CARTESIAN_POINT('Ctrl Pts',(0.25,1.5184626473304,0.968245836551854));
#14987=CARTESIAN_POINT('Ctrl Pts',(0.25,1.5815373526696,0.968245836551854));
#14988=CARTESIAN_POINT('Ctrl Pts',(0.243669763522488,1.61508042700263,0.969947158664211));
#14989=CARTESIAN_POINT('Ctrl Pts',(0.218115996279034,1.67663267125761,0.976011194447325));
#14990=CARTESIAN_POINT('Ctrl Pts',(0.198899276956455,1.70465411363682,0.980277651290853));
#14991=CARTESIAN_POINT('Ctrl Pts',(0.154657206767882,1.74889618382539,0.988223761669361));
#14992=CARTESIAN_POINT('Ctrl Pts',(0.126634476150511,1.76811531482682,0.992431259450842));
#14993=CARTESIAN_POINT('Ctrl Pts',(0.0650776639541239,1.79367084275751,
0.99835915024489));
#14994=CARTESIAN_POINT('Ctrl Pts',(0.0315329431858092,1.8,1.));
#14995=CARTESIAN_POINT('Ctrl Pts',(-0.0315329431858092,1.8,1.));
#14996=CARTESIAN_POINT('Ctrl Pts',(-0.0650776639541239,1.79367084275751,
0.99835915024489));
#14997=CARTESIAN_POINT('Ctrl Pts',(-0.126634476150511,1.76811531482682,
0.992431259450842));
#14998=CARTESIAN_POINT('Ctrl Pts',(-0.154657206767882,1.74889618382539,
0.988223761669361));
#14999=CARTESIAN_POINT('Ctrl Pts',(-0.198899276956455,1.70465411363682,
0.980277651290853));
#15000=CARTESIAN_POINT('Ctrl Pts',(-0.218115996279034,1.67663267125761,
0.976011194447325));
#15001=CARTESIAN_POINT('Ctrl Pts',(-0.243669763522489,1.61508042700263,
0.969947158664211));
#15002=CARTESIAN_POINT('Ctrl Pts',(-0.25,1.5815373526696,0.968245836551854));
#15003=CARTESIAN_POINT('Ctrl Pts',(-0.25,1.55,0.968245836551854));
#15004=CARTESIAN_POINT('',(-0.25,1.55,0.));
#15005=CARTESIAN_POINT('Origin',(1.65,2.25,0.));
#15006=CARTESIAN_POINT('',(-1.,2.25,-1.22464679914735E-16));
#15007=CARTESIAN_POINT('Origin',(0.,2.25,0.));
#15008=CARTESIAN_POINT('Origin',(1.75,0.85,0.));
#15009=CARTESIAN_POINT('',(-1.75,0.85,-2.14313189850787E-16));
#15010=CARTESIAN_POINT('Origin',(0.,0.85,0.));
#15011=CARTESIAN_POINT('Origin',(0.,0.,0.));
#15012=CARTESIAN_POINT('',(-1.75,-0.85,-2.14313189850787E-16));
#15013=CARTESIAN_POINT('Origin',(0.,-0.85,0.));
#15014=CARTESIAN_POINT('',(-1.75,0.,-2.14313189850787E-16));
#15015=CARTESIAN_POINT('Origin',(1.,-0.85,0.));
#15016=CARTESIAN_POINT('',(-1.,-0.85,-1.22464679914735E-16));
#15017=CARTESIAN_POINT('Origin',(0.,-0.85,0.));
#15018=CARTESIAN_POINT('Origin',(0.,0.7,0.));
#15019=CARTESIAN_POINT('',(-1.,0.7,-1.22464679914735E-16));
#17217=UNCERTAINTY_MEASURE_WITH_UNIT(LENGTH_MEASURE(0.001),#17323,
'DISTANCE_ACCURACY_VALUE',
'Maximum model space distance between geometric entities at asserted c
onnectivities');
#17261=UNCERTAINTY_MEASURE_WITH_UNIT(LENGTH_MEASURE(0.001),#17323,
'DISTANCE_ACCURACY_VALUE',
'Maximum model space distance between geometric entities at asserted c
onnectivities');
#17278=(
GEOMETRIC_REPRESENTATION_CONTEXT(3)
GLOBAL_UNCERTAINTY_ASSIGNED_CONTEXT((#17217))
GLOBAL_UNIT_ASSIGNED_CONTEXT((#17323,#17325,#17326))
REPRESENTATION_CONTEXT('','3D')
);
#17322=(
GEOMETRIC_REPRESENTATION_CONTEXT(3)
GLOBAL_UNCERTAINTY_ASSIGNED_CONTEXT((#17261))
GLOBAL_UNIT_ASSIGNED_CONTEXT((#17323,#17325,#17326))
REPRESENTATION_CONTEXT('','3D')
);
#17323=(
LENGTH_UNIT()
NAMED_UNIT(*)
SI_UNIT(.CENTI.,.METRE.)
);
#17325=(
NAMED_UNIT(*)
PLANE_ANGLE_UNIT()
SI_UNIT($,.RADIAN.)
);
#17326=(
NAMED_UNIT(*)
SI_UNIT($,.STERADIAN.)
SOLID_ANGLE_UNIT()
);
#17343=SHAPE_DEFINITION_REPRESENTATION(#17403,#17574);
#17403=PRODUCT_DEFINITION_SHAPE('',$,#17635);
#17574=SHAPE_REPRESENTATION('',(#10014),#17278);
#17618=PRODUCT_DEFINITION_CONTEXT('part definition',#17800,'design');
#17635=PRODUCT_DEFINITION('Insert bearing','Insert bearing',#17695,#17618);
#17695=PRODUCT_DEFINITION_FORMATION('',$,#17818);
#17800=APPLICATION_CONTEXT(
'Core Data for Automotive Mechanical Design Process');
#17801=PRODUCT_CONTEXT('part definition',#17800,'mechanical');
#17818=PRODUCT('Insert bearing','Insert bearing','Insert bearing',(#17801));
#17925=COLOUR_RGB('Grey',0.48,0.52,0.57);
#17926=FILL_AREA_STYLE_COLOUR('',#17925);
#17927=FILL_AREA_STYLE('',(#17926));
#17928=SURFACE_STYLE_FILL_AREA(#17927);
#17929=SURFACE_SIDE_STYLE('',(#17928));
#17930=SURFACE_STYLE_USAGE(.BOTH.,#17929);
#17931=PRESENTATION_STYLE_ASSIGNMENT((#17930));
ENDSEC;
END-ISO-10303-21;
